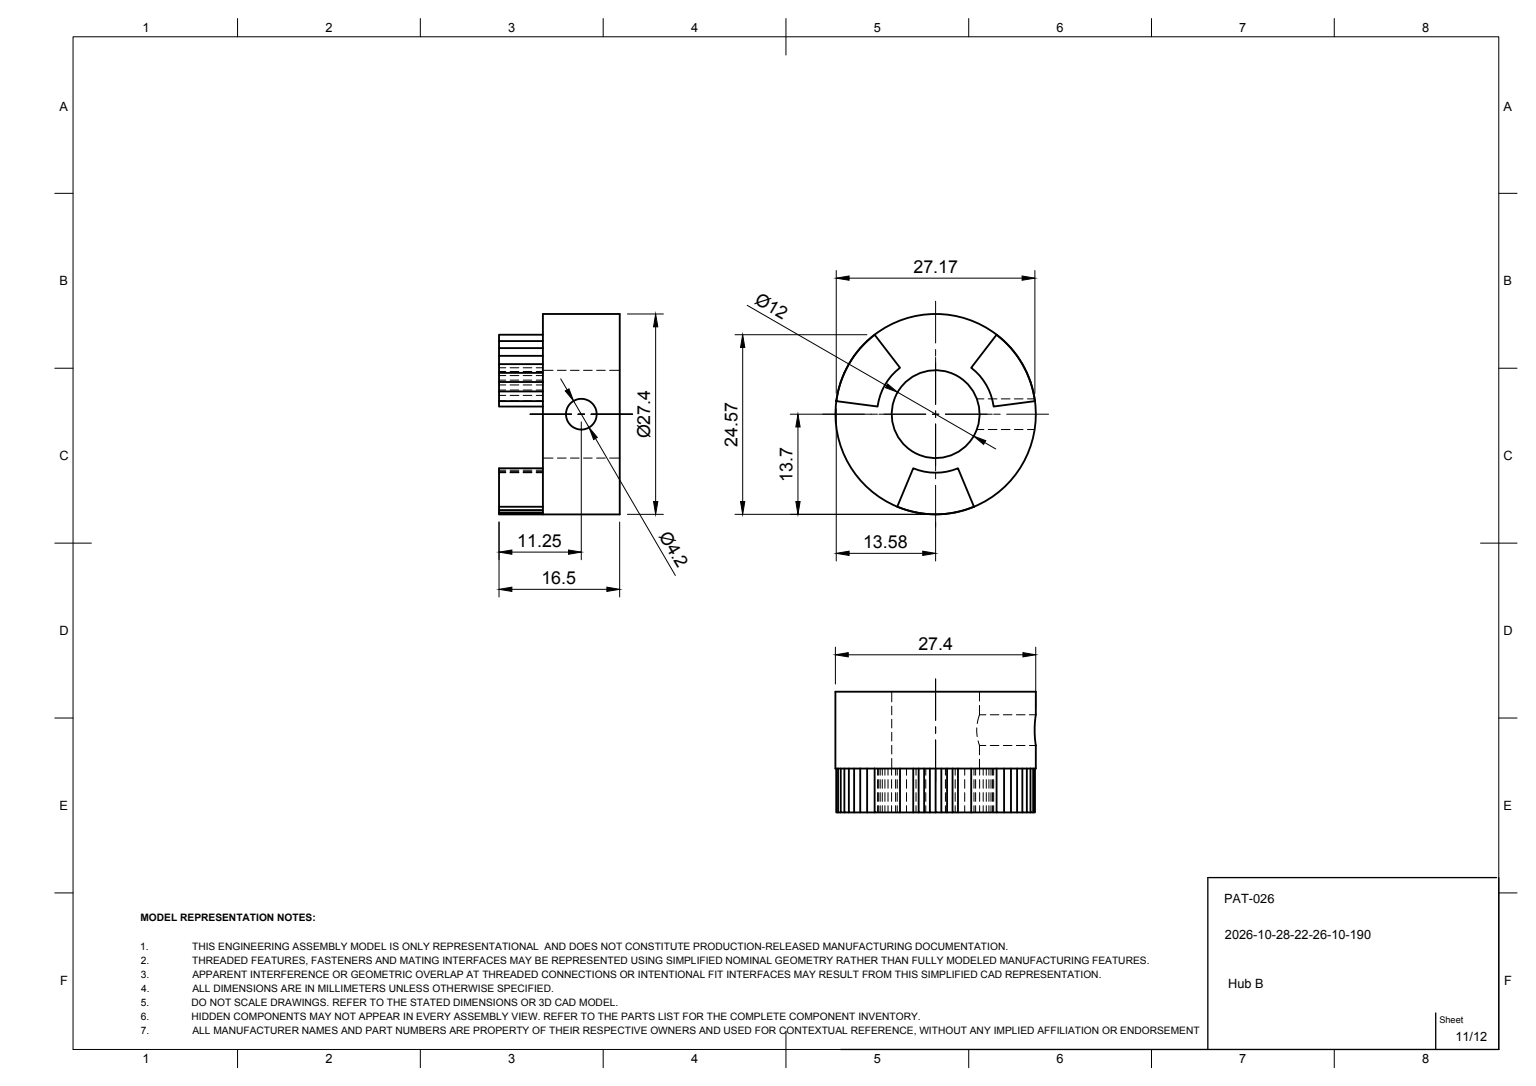
ISO-10303-21;
HEADER;
/* Generated by software containing ST-Developer
 * from STEP Tools, Inc. (www.steptools.com) 
 */

FILE_DESCRIPTION(
/* description */ ('PAT-026'),
/* implementation_level */ '2;1');

FILE_NAME(
/* name */ 'Hub B.step',
/* time_stamp */ '2026-10-28T22:25:58-07:00',
/* author */ (''),
/* organization */ (''),
/* preprocessor_version */ 'ST-DEVELOPER v20.2',
/* originating_system */ 'Autodesk Translation Framework v15.17.0.0',
/* authorisation */ '');

FILE_SCHEMA (('AUTOMOTIVE_DESIGN { 1 0 10303 214 3 1 1 }'));
ENDSEC;

DATA;
#10=MECHANICAL_DESIGN_GEOMETRIC_PRESENTATION_REPRESENTATION('',(#149),#12343);
#100=B_SPLINE_CURVE_WITH_KNOTS('',3,(#10943,#10944,#10945,#10946,#10947,
#10948,#10949,#10950,#10951,#10952,#10953,#10954,#10955,#10956,#10957,#10958,
#10959,#10960),.UNSPECIFIED.,.F.,.F.,(4,2,2,2,2,2,2,2,4),(0.,0.0798638474423531,
0.159727694884706,0.239545993340072,0.319364291795438,0.399182590250804,
0.47900088870617,0.558864736148523,0.638728583590876),.UNSPECIFIED.);
#101=B_SPLINE_CURVE_WITH_KNOTS('',3,(#10961,#10962,#10963,#10964,#10965,
#10966,#10967,#10968,#10969,#10970,#10971,#10972,#10973,#10974,#10975,#10976,
#10977,#10978),.UNSPECIFIED.,.F.,.F.,(4,2,2,2,2,2,2,2,4),(0.638728583590876,
0.718592431033229,0.798456278475583,0.878274576930949,0.958092875386314,
1.03791117384168,1.11772947229705,1.1975933197394,1.27745716718175),
 .UNSPECIFIED.);
#102=B_SPLINE_CURVE_WITH_KNOTS('',3,(#10982,#10983,#10984,#10985,#10986,
#10987,#10988,#10989,#10990,#10991,#10992,#10993,#10994,#10995,#10996,#10997,
#10998,#10999),.UNSPECIFIED.,.F.,.F.,(4,2,2,2,2,2,2,2,4),(0.,0.079239302416133,
0.158478604832266,0.237716399152057,0.316954193471848,0.39619198779164,
0.475429782111431,0.554669084527564,0.633908386943697),.UNSPECIFIED.);
#103=B_SPLINE_CURVE_WITH_KNOTS('',3,(#11000,#11001,#11002,#11003,#11004,
#11005,#11006,#11007,#11008,#11009,#11010,#11011,#11012,#11013,#11014,#11015,
#11016,#11017),.UNSPECIFIED.,.F.,.F.,(4,2,2,2,2,2,2,2,4),(0.633908386943697,
0.71314768935983,0.792386991775963,0.871624786095754,0.950862580415545,
1.03010037473534,1.10933816905513,1.18857747147126,1.26781677388739),
 .UNSPECIFIED.);
#127=SHAPE_REPRESENTATION_RELATIONSHIP('SRR','None',#12405,#138);
#138=ADVANCED_BREP_SHAPE_REPRESENTATION('',(#158),#12340);
#149=STYLED_ITEM('',(#12526),#158);
#158=MANIFOLD_SOLID_BREP('Body1',#7357);
#189=FACE_BOUND('',#1151,.T.);
#190=FACE_BOUND('',#1178,.T.);
#191=FACE_BOUND('',#1236,.T.);
#192=FACE_BOUND('',#1238,.T.);
#327=PLANE('',#7740);
#328=PLANE('',#7741);
#329=PLANE('',#7742);
#330=PLANE('',#7743);
#331=PLANE('',#7744);
#332=PLANE('',#7745);
#333=PLANE('',#7746);
#334=PLANE('',#7747);
#335=PLANE('',#7748);
#336=PLANE('',#7749);
#337=PLANE('',#7750);
#338=PLANE('',#7751);
#339=PLANE('',#7752);
#340=PLANE('',#7753);
#341=PLANE('',#7754);
#342=PLANE('',#7755);
#343=PLANE('',#7756);
#344=PLANE('',#7757);
#345=PLANE('',#7758);
#346=PLANE('',#7759);
#347=PLANE('',#7761);
#348=PLANE('',#7763);
#349=PLANE('',#7765);
#350=PLANE('',#7767);
#351=PLANE('',#7769);
#352=PLANE('',#7771);
#353=PLANE('',#7776);
#354=PLANE('',#7778);
#355=PLANE('',#7780);
#356=PLANE('',#7781);
#357=PLANE('',#7782);
#358=PLANE('',#7783);
#359=PLANE('',#7784);
#360=PLANE('',#7785);
#361=PLANE('',#7786);
#362=PLANE('',#7787);
#363=PLANE('',#7788);
#364=PLANE('',#7789);
#365=PLANE('',#7790);
#366=PLANE('',#7791);
#367=PLANE('',#7792);
#368=PLANE('',#7793);
#369=PLANE('',#7794);
#370=PLANE('',#7795);
#371=PLANE('',#7796);
#372=PLANE('',#7797);
#373=PLANE('',#7798);
#374=PLANE('',#7799);
#375=PLANE('',#7801);
#376=PLANE('',#7803);
#377=PLANE('',#7805);
#378=PLANE('',#7807);
#379=PLANE('',#7809);
#380=PLANE('',#7811);
#381=PLANE('',#7813);
#382=PLANE('',#7815);
#383=PLANE('',#7816);
#384=PLANE('',#7817);
#385=PLANE('',#7818);
#386=PLANE('',#7819);
#387=PLANE('',#7820);
#388=PLANE('',#7821);
#389=PLANE('',#7822);
#390=PLANE('',#7823);
#391=PLANE('',#7824);
#392=PLANE('',#7825);
#393=PLANE('',#7826);
#394=PLANE('',#7827);
#395=PLANE('',#7828);
#396=PLANE('',#7829);
#397=PLANE('',#7830);
#398=PLANE('',#7831);
#399=PLANE('',#7832);
#400=PLANE('',#7833);
#401=PLANE('',#7834);
#402=PLANE('',#7836);
#403=PLANE('',#7838);
#404=PLANE('',#7840);
#405=PLANE('',#7842);
#406=PLANE('',#7844);
#407=PLANE('',#7846);
#408=PLANE('',#7848);
#409=PLANE('',#7852);
#718=FACE_OUTER_BOUND('',#1149,.T.);
#719=FACE_OUTER_BOUND('',#1150,.T.);
#720=FACE_OUTER_BOUND('',#1152,.T.);
#721=FACE_OUTER_BOUND('',#1153,.T.);
#722=FACE_OUTER_BOUND('',#1154,.T.);
#723=FACE_OUTER_BOUND('',#1155,.T.);
#724=FACE_OUTER_BOUND('',#1156,.T.);
#725=FACE_OUTER_BOUND('',#1157,.T.);
#726=FACE_OUTER_BOUND('',#1158,.T.);
#727=FACE_OUTER_BOUND('',#1159,.T.);
#728=FACE_OUTER_BOUND('',#1160,.T.);
#729=FACE_OUTER_BOUND('',#1161,.T.);
#730=FACE_OUTER_BOUND('',#1162,.T.);
#731=FACE_OUTER_BOUND('',#1163,.T.);
#732=FACE_OUTER_BOUND('',#1164,.T.);
#733=FACE_OUTER_BOUND('',#1165,.T.);
#734=FACE_OUTER_BOUND('',#1166,.T.);
#735=FACE_OUTER_BOUND('',#1167,.T.);
#736=FACE_OUTER_BOUND('',#1168,.T.);
#737=FACE_OUTER_BOUND('',#1169,.T.);
#738=FACE_OUTER_BOUND('',#1170,.T.);
#739=FACE_OUTER_BOUND('',#1171,.T.);
#740=FACE_OUTER_BOUND('',#1172,.T.);
#741=FACE_OUTER_BOUND('',#1173,.T.);
#742=FACE_OUTER_BOUND('',#1174,.T.);
#743=FACE_OUTER_BOUND('',#1175,.T.);
#744=FACE_OUTER_BOUND('',#1176,.T.);
#745=FACE_OUTER_BOUND('',#1177,.T.);
#746=FACE_OUTER_BOUND('',#1179,.T.);
#747=FACE_OUTER_BOUND('',#1180,.T.);
#748=FACE_OUTER_BOUND('',#1181,.T.);
#749=FACE_OUTER_BOUND('',#1182,.T.);
#750=FACE_OUTER_BOUND('',#1183,.T.);
#751=FACE_OUTER_BOUND('',#1184,.T.);
#752=FACE_OUTER_BOUND('',#1185,.T.);
#753=FACE_OUTER_BOUND('',#1186,.T.);
#754=FACE_OUTER_BOUND('',#1187,.T.);
#755=FACE_OUTER_BOUND('',#1188,.T.);
#756=FACE_OUTER_BOUND('',#1189,.T.);
#757=FACE_OUTER_BOUND('',#1190,.T.);
#758=FACE_OUTER_BOUND('',#1191,.T.);
#759=FACE_OUTER_BOUND('',#1192,.T.);
#760=FACE_OUTER_BOUND('',#1193,.T.);
#761=FACE_OUTER_BOUND('',#1194,.T.);
#762=FACE_OUTER_BOUND('',#1195,.T.);
#763=FACE_OUTER_BOUND('',#1196,.T.);
#764=FACE_OUTER_BOUND('',#1197,.T.);
#765=FACE_OUTER_BOUND('',#1198,.T.);
#766=FACE_OUTER_BOUND('',#1199,.T.);
#767=FACE_OUTER_BOUND('',#1200,.T.);
#768=FACE_OUTER_BOUND('',#1201,.T.);
#769=FACE_OUTER_BOUND('',#1202,.T.);
#770=FACE_OUTER_BOUND('',#1203,.T.);
#771=FACE_OUTER_BOUND('',#1204,.T.);
#772=FACE_OUTER_BOUND('',#1205,.T.);
#773=FACE_OUTER_BOUND('',#1206,.T.);
#774=FACE_OUTER_BOUND('',#1207,.T.);
#775=FACE_OUTER_BOUND('',#1208,.T.);
#776=FACE_OUTER_BOUND('',#1209,.T.);
#777=FACE_OUTER_BOUND('',#1210,.T.);
#778=FACE_OUTER_BOUND('',#1211,.T.);
#779=FACE_OUTER_BOUND('',#1212,.T.);
#780=FACE_OUTER_BOUND('',#1213,.T.);
#781=FACE_OUTER_BOUND('',#1214,.T.);
#782=FACE_OUTER_BOUND('',#1215,.T.);
#783=FACE_OUTER_BOUND('',#1216,.T.);
#784=FACE_OUTER_BOUND('',#1217,.T.);
#785=FACE_OUTER_BOUND('',#1218,.T.);
#786=FACE_OUTER_BOUND('',#1219,.T.);
#787=FACE_OUTER_BOUND('',#1220,.T.);
#788=FACE_OUTER_BOUND('',#1221,.T.);
#789=FACE_OUTER_BOUND('',#1222,.T.);
#790=FACE_OUTER_BOUND('',#1223,.T.);
#791=FACE_OUTER_BOUND('',#1224,.T.);
#792=FACE_OUTER_BOUND('',#1225,.T.);
#793=FACE_OUTER_BOUND('',#1226,.T.);
#794=FACE_OUTER_BOUND('',#1227,.T.);
#795=FACE_OUTER_BOUND('',#1228,.T.);
#796=FACE_OUTER_BOUND('',#1229,.T.);
#797=FACE_OUTER_BOUND('',#1230,.T.);
#798=FACE_OUTER_BOUND('',#1231,.T.);
#799=FACE_OUTER_BOUND('',#1232,.T.);
#800=FACE_OUTER_BOUND('',#1233,.T.);
#801=FACE_OUTER_BOUND('',#1234,.T.);
#802=FACE_OUTER_BOUND('',#1235,.T.);
#803=FACE_OUTER_BOUND('',#1237,.T.);
#1149=EDGE_LOOP('',(#5633,#5634,#5635,#5636,#5637,#5638));
#1150=EDGE_LOOP('',(#5639,#5640,#5641,#5642));
#1151=EDGE_LOOP('',(#5643,#5644));
#1152=EDGE_LOOP('',(#5645,#5646,#5647,#5648));
#1153=EDGE_LOOP('',(#5649,#5650,#5651,#5652));
#1154=EDGE_LOOP('',(#5653,#5654,#5655,#5656));
#1155=EDGE_LOOP('',(#5657,#5658,#5659,#5660));
#1156=EDGE_LOOP('',(#5661,#5662,#5663,#5664));
#1157=EDGE_LOOP('',(#5665,#5666,#5667,#5668));
#1158=EDGE_LOOP('',(#5669,#5670,#5671,#5672));
#1159=EDGE_LOOP('',(#5673,#5674,#5675,#5676));
#1160=EDGE_LOOP('',(#5677,#5678,#5679,#5680));
#1161=EDGE_LOOP('',(#5681,#5682,#5683,#5684));
#1162=EDGE_LOOP('',(#5685,#5686,#5687,#5688));
#1163=EDGE_LOOP('',(#5689,#5690,#5691,#5692));
#1164=EDGE_LOOP('',(#5693,#5694,#5695,#5696));
#1165=EDGE_LOOP('',(#5697,#5698,#5699,#5700));
#1166=EDGE_LOOP('',(#5701,#5702,#5703,#5704));
#1167=EDGE_LOOP('',(#5705,#5706,#5707,#5708));
#1168=EDGE_LOOP('',(#5709,#5710,#5711,#5712));
#1169=EDGE_LOOP('',(#5713,#5714,#5715,#5716));
#1170=EDGE_LOOP('',(#5717,#5718,#5719,#5720,#5721,#5722,#5723,#5724,#5725,
#5726,#5727,#5728,#5729,#5730,#5731,#5732,#5733,#5734));
#1171=EDGE_LOOP('',(#5735,#5736));
#1172=EDGE_LOOP('',(#5737,#5738));
#1173=EDGE_LOOP('',(#5739,#5740));
#1174=EDGE_LOOP('',(#5741,#5742));
#1175=EDGE_LOOP('',(#5743,#5744));
#1176=EDGE_LOOP('',(#5745,#5746));
#1177=EDGE_LOOP('',(#5747,#5748,#5749,#5750,#5751,#5752,#5753,#5754,#5755,
#5756,#5757,#5758,#5759,#5760,#5761,#5762,#5763,#5764,#5765,#5766,#5767,
#5768,#5769,#5770,#5771,#5772,#5773,#5774,#5775,#5776,#5777,#5778,#5779,
#5780));
#1178=EDGE_LOOP('',(#5781));
#1179=EDGE_LOOP('',(#5782,#5783));
#1180=EDGE_LOOP('',(#5784,#5785));
#1181=EDGE_LOOP('',(#5786,#5787,#5788,#5789));
#1182=EDGE_LOOP('',(#5790,#5791,#5792,#5793));
#1183=EDGE_LOOP('',(#5794,#5795,#5796,#5797));
#1184=EDGE_LOOP('',(#5798,#5799,#5800,#5801));
#1185=EDGE_LOOP('',(#5802,#5803,#5804,#5805));
#1186=EDGE_LOOP('',(#5806,#5807,#5808,#5809));
#1187=EDGE_LOOP('',(#5810,#5811,#5812,#5813));
#1188=EDGE_LOOP('',(#5814,#5815,#5816,#5817));
#1189=EDGE_LOOP('',(#5818,#5819,#5820,#5821));
#1190=EDGE_LOOP('',(#5822,#5823,#5824,#5825));
#1191=EDGE_LOOP('',(#5826,#5827,#5828,#5829));
#1192=EDGE_LOOP('',(#5830,#5831,#5832,#5833));
#1193=EDGE_LOOP('',(#5834,#5835,#5836,#5837));
#1194=EDGE_LOOP('',(#5838,#5839,#5840,#5841));
#1195=EDGE_LOOP('',(#5842,#5843,#5844,#5845));
#1196=EDGE_LOOP('',(#5846,#5847,#5848,#5849));
#1197=EDGE_LOOP('',(#5850,#5851,#5852,#5853));
#1198=EDGE_LOOP('',(#5854,#5855,#5856,#5857));
#1199=EDGE_LOOP('',(#5858,#5859,#5860,#5861,#5862,#5863,#5864,#5865,#5866,
#5867,#5868,#5869,#5870,#5871,#5872,#5873,#5874,#5875));
#1200=EDGE_LOOP('',(#5876,#5877));
#1201=EDGE_LOOP('',(#5878,#5879));
#1202=EDGE_LOOP('',(#5880,#5881));
#1203=EDGE_LOOP('',(#5882,#5883));
#1204=EDGE_LOOP('',(#5884,#5885));
#1205=EDGE_LOOP('',(#5886,#5887));
#1206=EDGE_LOOP('',(#5888,#5889));
#1207=EDGE_LOOP('',(#5890,#5891));
#1208=EDGE_LOOP('',(#5892,#5893,#5894,#5895));
#1209=EDGE_LOOP('',(#5896,#5897,#5898,#5899));
#1210=EDGE_LOOP('',(#5900,#5901,#5902,#5903));
#1211=EDGE_LOOP('',(#5904,#5905,#5906,#5907));
#1212=EDGE_LOOP('',(#5908,#5909,#5910,#5911));
#1213=EDGE_LOOP('',(#5912,#5913,#5914,#5915));
#1214=EDGE_LOOP('',(#5916,#5917,#5918,#5919));
#1215=EDGE_LOOP('',(#5920,#5921,#5922,#5923));
#1216=EDGE_LOOP('',(#5924,#5925,#5926,#5927));
#1217=EDGE_LOOP('',(#5928,#5929,#5930,#5931));
#1218=EDGE_LOOP('',(#5932,#5933,#5934,#5935));
#1219=EDGE_LOOP('',(#5936,#5937,#5938,#5939));
#1220=EDGE_LOOP('',(#5940,#5941,#5942,#5943));
#1221=EDGE_LOOP('',(#5944,#5945,#5946,#5947));
#1222=EDGE_LOOP('',(#5948,#5949,#5950,#5951));
#1223=EDGE_LOOP('',(#5952,#5953,#5954,#5955));
#1224=EDGE_LOOP('',(#5956,#5957,#5958,#5959));
#1225=EDGE_LOOP('',(#5960,#5961,#5962,#5963));
#1226=EDGE_LOOP('',(#5964,#5965,#5966,#5967,#5968,#5969,#5970,#5971,#5972,
#5973,#5974,#5975,#5976,#5977,#5978,#5979,#5980,#5981));
#1227=EDGE_LOOP('',(#5982,#5983));
#1228=EDGE_LOOP('',(#5984,#5985));
#1229=EDGE_LOOP('',(#5986,#5987));
#1230=EDGE_LOOP('',(#5988,#5989));
#1231=EDGE_LOOP('',(#5990,#5991));
#1232=EDGE_LOOP('',(#5992,#5993));
#1233=EDGE_LOOP('',(#5994,#5995));
#1234=EDGE_LOOP('',(#5996,#5997));
#1235=EDGE_LOOP('',(#5998,#5999,#6000,#6001,#6002,#6003,#6004,#6005,#6006,
#6007,#6008,#6009,#6010,#6011,#6012,#6013,#6014,#6015,#6016,#6017,#6018,
#6019,#6020,#6021,#6022,#6023,#6024,#6025,#6026,#6027,#6028));
#1236=EDGE_LOOP('',(#6029,#6030));
#1237=EDGE_LOOP('',(#6031));
#1238=EDGE_LOOP('',(#6032));
#1676=LINE('',#10980,#2548);
#1677=LINE('',#11022,#2549);
#1678=LINE('',#11027,#2550);
#1679=LINE('',#11029,#2551);
#1680=LINE('',#11031,#2552);
#1681=LINE('',#11032,#2553);
#1682=LINE('',#11035,#2554);
#1683=LINE('',#11037,#2555);
#1684=LINE('',#11038,#2556);
#1685=LINE('',#11041,#2557);
#1686=LINE('',#11043,#2558);
#1687=LINE('',#11044,#2559);
#1688=LINE('',#11047,#2560);
#1689=LINE('',#11049,#2561);
#1690=LINE('',#11050,#2562);
#1691=LINE('',#11053,#2563);
#1692=LINE('',#11055,#2564);
#1693=LINE('',#11056,#2565);
#1694=LINE('',#11059,#2566);
#1695=LINE('',#11061,#2567);
#1696=LINE('',#11062,#2568);
#1697=LINE('',#11065,#2569);
#1698=LINE('',#11067,#2570);
#1699=LINE('',#11068,#2571);
#1700=LINE('',#11071,#2572);
#1701=LINE('',#11073,#2573);
#1702=LINE('',#11074,#2574);
#1703=LINE('',#11077,#2575);
#1704=LINE('',#11079,#2576);
#1705=LINE('',#11080,#2577);
#1706=LINE('',#11083,#2578);
#1707=LINE('',#11085,#2579);
#1708=LINE('',#11086,#2580);
#1709=LINE('',#11089,#2581);
#1710=LINE('',#11091,#2582);
#1711=LINE('',#11092,#2583);
#1712=LINE('',#11095,#2584);
#1713=LINE('',#11097,#2585);
#1714=LINE('',#11098,#2586);
#1715=LINE('',#11101,#2587);
#1716=LINE('',#11103,#2588);
#1717=LINE('',#11104,#2589);
#1718=LINE('',#11107,#2590);
#1719=LINE('',#11109,#2591);
#1720=LINE('',#11110,#2592);
#1721=LINE('',#11113,#2593);
#1722=LINE('',#11115,#2594);
#1723=LINE('',#11116,#2595);
#1724=LINE('',#11119,#2596);
#1725=LINE('',#11121,#2597);
#1726=LINE('',#11122,#2598);
#1727=LINE('',#11125,#2599);
#1728=LINE('',#11127,#2600);
#1729=LINE('',#11128,#2601);
#1730=LINE('',#11130,#2602);
#1731=LINE('',#11131,#2603);
#1732=LINE('',#11151,#2604);
#1733=LINE('',#11153,#2605);
#1734=LINE('',#11155,#2606);
#1735=LINE('',#11157,#2607);
#1736=LINE('',#11159,#2608);
#1737=LINE('',#11161,#2609);
#1738=LINE('',#11163,#2610);
#1739=LINE('',#11165,#2611);
#1740=LINE('',#11167,#2612);
#1741=LINE('',#11169,#2613);
#1742=LINE('',#11173,#2614);
#1743=LINE('',#11175,#2615);
#1744=LINE('',#11177,#2616);
#1745=LINE('',#11179,#2617);
#1746=LINE('',#11181,#2618);
#1747=LINE('',#11183,#2619);
#1748=LINE('',#11185,#2620);
#1749=LINE('',#11187,#2621);
#1750=LINE('',#11189,#2622);
#1751=LINE('',#11191,#2623);
#1752=LINE('',#11200,#2624);
#1753=LINE('',#11201,#2625);
#1754=LINE('',#11202,#2626);
#1755=LINE('',#11205,#2627);
#1756=LINE('',#11206,#2628);
#1757=LINE('',#11209,#2629);
#1758=LINE('',#11210,#2630);
#1759=LINE('',#11213,#2631);
#1760=LINE('',#11214,#2632);
#1761=LINE('',#11217,#2633);
#1762=LINE('',#11218,#2634);
#1763=LINE('',#11221,#2635);
#1764=LINE('',#11222,#2636);
#1765=LINE('',#11225,#2637);
#1766=LINE('',#11226,#2638);
#1767=LINE('',#11229,#2639);
#1768=LINE('',#11230,#2640);
#1769=LINE('',#11233,#2641);
#1770=LINE('',#11234,#2642);
#1771=LINE('',#11237,#2643);
#1772=LINE('',#11239,#2644);
#1773=LINE('',#11240,#2645);
#1774=LINE('',#11243,#2646);
#1775=LINE('',#11245,#2647);
#1776=LINE('',#11246,#2648);
#1777=LINE('',#11249,#2649);
#1778=LINE('',#11251,#2650);
#1779=LINE('',#11252,#2651);
#1780=LINE('',#11255,#2652);
#1781=LINE('',#11257,#2653);
#1782=LINE('',#11258,#2654);
#1783=LINE('',#11261,#2655);
#1784=LINE('',#11263,#2656);
#1785=LINE('',#11264,#2657);
#1786=LINE('',#11267,#2658);
#1787=LINE('',#11269,#2659);
#1788=LINE('',#11270,#2660);
#1789=LINE('',#11273,#2661);
#1790=LINE('',#11275,#2662);
#1791=LINE('',#11276,#2663);
#1792=LINE('',#11279,#2664);
#1793=LINE('',#11280,#2665);
#1794=LINE('',#11281,#2666);
#1795=LINE('',#11283,#2667);
#1796=LINE('',#11304,#2668);
#1797=LINE('',#11305,#2669);
#1798=LINE('',#11306,#2670);
#1799=LINE('',#11309,#2671);
#1800=LINE('',#11310,#2672);
#1801=LINE('',#11313,#2673);
#1802=LINE('',#11314,#2674);
#1803=LINE('',#11317,#2675);
#1804=LINE('',#11318,#2676);
#1805=LINE('',#11321,#2677);
#1806=LINE('',#11322,#2678);
#1807=LINE('',#11325,#2679);
#1808=LINE('',#11326,#2680);
#1809=LINE('',#11329,#2681);
#1810=LINE('',#11330,#2682);
#1811=LINE('',#11333,#2683);
#1812=LINE('',#11334,#2684);
#1813=LINE('',#11337,#2685);
#1814=LINE('',#11338,#2686);
#1815=LINE('',#11341,#2687);
#1816=LINE('',#11343,#2688);
#1817=LINE('',#11344,#2689);
#1818=LINE('',#11347,#2690);
#1819=LINE('',#11349,#2691);
#1820=LINE('',#11350,#2692);
#1821=LINE('',#11353,#2693);
#1822=LINE('',#11355,#2694);
#1823=LINE('',#11356,#2695);
#1824=LINE('',#11359,#2696);
#1825=LINE('',#11361,#2697);
#1826=LINE('',#11362,#2698);
#1827=LINE('',#11365,#2699);
#1828=LINE('',#11367,#2700);
#1829=LINE('',#11368,#2701);
#1830=LINE('',#11371,#2702);
#1831=LINE('',#11373,#2703);
#1832=LINE('',#11374,#2704);
#1833=LINE('',#11377,#2705);
#1834=LINE('',#11379,#2706);
#1835=LINE('',#11380,#2707);
#1836=LINE('',#11383,#2708);
#1837=LINE('',#11384,#2709);
#1838=LINE('',#11385,#2710);
#1839=LINE('',#11387,#2711);
#1840=LINE('',#11408,#2712);
#2548=VECTOR('',#8838,0.21);
#2549=VECTOR('',#8843,0.6);
#2550=VECTOR('',#8848,1.);
#2551=VECTOR('',#8849,1.);
#2552=VECTOR('',#8850,1.);
#2553=VECTOR('',#8851,1.);
#2554=VECTOR('',#8854,1.);
#2555=VECTOR('',#8855,1.);
#2556=VECTOR('',#8856,1.);
#2557=VECTOR('',#8859,1.);
#2558=VECTOR('',#8860,1.);
#2559=VECTOR('',#8861,1.);
#2560=VECTOR('',#8864,1.);
#2561=VECTOR('',#8865,1.);
#2562=VECTOR('',#8866,1.);
#2563=VECTOR('',#8869,1.);
#2564=VECTOR('',#8870,1.);
#2565=VECTOR('',#8871,1.);
#2566=VECTOR('',#8874,1.);
#2567=VECTOR('',#8875,1.);
#2568=VECTOR('',#8876,1.);
#2569=VECTOR('',#8879,1.);
#2570=VECTOR('',#8880,1.);
#2571=VECTOR('',#8881,1.);
#2572=VECTOR('',#8884,1.);
#2573=VECTOR('',#8885,1.);
#2574=VECTOR('',#8886,1.);
#2575=VECTOR('',#8889,1.);
#2576=VECTOR('',#8890,1.);
#2577=VECTOR('',#8891,1.);
#2578=VECTOR('',#8894,1.);
#2579=VECTOR('',#8895,1.);
#2580=VECTOR('',#8896,1.);
#2581=VECTOR('',#8899,1.);
#2582=VECTOR('',#8900,1.);
#2583=VECTOR('',#8901,1.);
#2584=VECTOR('',#8904,1.);
#2585=VECTOR('',#8905,1.);
#2586=VECTOR('',#8906,1.);
#2587=VECTOR('',#8909,1.);
#2588=VECTOR('',#8910,1.);
#2589=VECTOR('',#8911,1.);
#2590=VECTOR('',#8914,1.);
#2591=VECTOR('',#8915,1.);
#2592=VECTOR('',#8916,1.);
#2593=VECTOR('',#8919,1.);
#2594=VECTOR('',#8920,1.);
#2595=VECTOR('',#8921,1.);
#2596=VECTOR('',#8924,1.);
#2597=VECTOR('',#8925,1.);
#2598=VECTOR('',#8926,1.);
#2599=VECTOR('',#8929,1.);
#2600=VECTOR('',#8930,1.);
#2601=VECTOR('',#8931,1.);
#2602=VECTOR('',#8934,1.);
#2603=VECTOR('',#8935,1.);
#2604=VECTOR('',#8968,1.);
#2605=VECTOR('',#8969,1.);
#2606=VECTOR('',#8970,1.);
#2607=VECTOR('',#8971,1.);
#2608=VECTOR('',#8972,1.);
#2609=VECTOR('',#8973,1.);
#2610=VECTOR('',#8974,1.);
#2611=VECTOR('',#8975,1.);
#2612=VECTOR('',#8976,1.);
#2613=VECTOR('',#8977,1.);
#2614=VECTOR('',#8980,1.);
#2615=VECTOR('',#8981,1.);
#2616=VECTOR('',#8982,1.);
#2617=VECTOR('',#8983,1.);
#2618=VECTOR('',#8984,1.);
#2619=VECTOR('',#8985,1.);
#2620=VECTOR('',#8986,1.);
#2621=VECTOR('',#8987,1.);
#2622=VECTOR('',#8988,1.);
#2623=VECTOR('',#8989,1.);
#2624=VECTOR('',#9002,1.);
#2625=VECTOR('',#9003,1.);
#2626=VECTOR('',#9004,1.);
#2627=VECTOR('',#9007,1.);
#2628=VECTOR('',#9008,1.);
#2629=VECTOR('',#9011,1.);
#2630=VECTOR('',#9012,1.);
#2631=VECTOR('',#9015,1.);
#2632=VECTOR('',#9016,1.);
#2633=VECTOR('',#9019,1.);
#2634=VECTOR('',#9020,1.);
#2635=VECTOR('',#9023,1.);
#2636=VECTOR('',#9024,1.);
#2637=VECTOR('',#9027,1.);
#2638=VECTOR('',#9028,1.);
#2639=VECTOR('',#9031,1.);
#2640=VECTOR('',#9032,1.);
#2641=VECTOR('',#9035,1.);
#2642=VECTOR('',#9036,1.);
#2643=VECTOR('',#9039,1.);
#2644=VECTOR('',#9040,1.);
#2645=VECTOR('',#9041,1.);
#2646=VECTOR('',#9044,1.);
#2647=VECTOR('',#9045,1.);
#2648=VECTOR('',#9046,1.);
#2649=VECTOR('',#9049,1.);
#2650=VECTOR('',#9050,1.);
#2651=VECTOR('',#9051,1.);
#2652=VECTOR('',#9054,1.);
#2653=VECTOR('',#9055,1.);
#2654=VECTOR('',#9056,1.);
#2655=VECTOR('',#9059,1.);
#2656=VECTOR('',#9060,1.);
#2657=VECTOR('',#9061,1.);
#2658=VECTOR('',#9064,1.);
#2659=VECTOR('',#9065,1.);
#2660=VECTOR('',#9066,1.);
#2661=VECTOR('',#9069,1.);
#2662=VECTOR('',#9070,1.);
#2663=VECTOR('',#9071,1.);
#2664=VECTOR('',#9074,1.);
#2665=VECTOR('',#9075,1.);
#2666=VECTOR('',#9076,1.);
#2667=VECTOR('',#9079,1.);
#2668=VECTOR('',#9116,1.);
#2669=VECTOR('',#9117,1.);
#2670=VECTOR('',#9118,1.);
#2671=VECTOR('',#9121,1.);
#2672=VECTOR('',#9122,1.);
#2673=VECTOR('',#9125,1.);
#2674=VECTOR('',#9126,1.);
#2675=VECTOR('',#9129,1.);
#2676=VECTOR('',#9130,1.);
#2677=VECTOR('',#9133,1.);
#2678=VECTOR('',#9134,1.);
#2679=VECTOR('',#9137,1.);
#2680=VECTOR('',#9138,1.);
#2681=VECTOR('',#9141,1.);
#2682=VECTOR('',#9142,1.);
#2683=VECTOR('',#9145,1.);
#2684=VECTOR('',#9146,1.);
#2685=VECTOR('',#9149,1.);
#2686=VECTOR('',#9150,1.);
#2687=VECTOR('',#9153,1.);
#2688=VECTOR('',#9154,1.);
#2689=VECTOR('',#9155,1.);
#2690=VECTOR('',#9158,1.);
#2691=VECTOR('',#9159,1.);
#2692=VECTOR('',#9160,1.);
#2693=VECTOR('',#9163,1.);
#2694=VECTOR('',#9164,1.);
#2695=VECTOR('',#9165,1.);
#2696=VECTOR('',#9168,1.);
#2697=VECTOR('',#9169,1.);
#2698=VECTOR('',#9170,1.);
#2699=VECTOR('',#9173,1.);
#2700=VECTOR('',#9174,1.);
#2701=VECTOR('',#9175,1.);
#2702=VECTOR('',#9178,1.);
#2703=VECTOR('',#9179,1.);
#2704=VECTOR('',#9180,1.);
#2705=VECTOR('',#9183,1.);
#2706=VECTOR('',#9184,1.);
#2707=VECTOR('',#9185,1.);
#2708=VECTOR('',#9188,1.);
#2709=VECTOR('',#9189,1.);
#2710=VECTOR('',#9190,1.);
#2711=VECTOR('',#9193,1.);
#2712=VECTOR('',#9232,1.37);
#3214=CIRCLE('',#7738,0.6);
#3215=CIRCLE('',#7739,0.6);
#3216=CIRCLE('',#7760,1.37);
#3217=CIRCLE('',#7762,1.37);
#3218=CIRCLE('',#7764,1.37);
#3219=CIRCLE('',#7766,1.37);
#3220=CIRCLE('',#7768,1.37);
#3221=CIRCLE('',#7770,1.37);
#3222=CIRCLE('',#7772,1.37);
#3223=CIRCLE('',#7773,1.37);
#3224=CIRCLE('',#7774,1.37);
#3225=CIRCLE('',#7775,1.37);
#3226=CIRCLE('',#7777,1.37);
#3227=CIRCLE('',#7779,1.37);
#3228=CIRCLE('',#7800,1.37);
#3229=CIRCLE('',#7802,1.37);
#3230=CIRCLE('',#7804,1.37);
#3231=CIRCLE('',#7806,1.37);
#3232=CIRCLE('',#7808,1.37);
#3233=CIRCLE('',#7810,1.37);
#3234=CIRCLE('',#7812,1.37);
#3235=CIRCLE('',#7814,1.37);
#3236=CIRCLE('',#7835,1.37);
#3237=CIRCLE('',#7837,1.37);
#3238=CIRCLE('',#7839,1.37);
#3239=CIRCLE('',#7841,1.37);
#3240=CIRCLE('',#7843,1.37);
#3241=CIRCLE('',#7845,1.37);
#3242=CIRCLE('',#7847,1.37);
#3243=CIRCLE('',#7849,1.37);
#3244=CIRCLE('',#7851,1.37);
#3485=VERTEX_POINT('',#10941);
#3486=VERTEX_POINT('',#10942);
#3487=VERTEX_POINT('',#10979);
#3488=VERTEX_POINT('',#10981);
#3489=VERTEX_POINT('',#11019);
#3490=VERTEX_POINT('',#11021);
#3491=VERTEX_POINT('',#11025);
#3492=VERTEX_POINT('',#11026);
#3493=VERTEX_POINT('',#11028);
#3494=VERTEX_POINT('',#11030);
#3495=VERTEX_POINT('',#11034);
#3496=VERTEX_POINT('',#11036);
#3497=VERTEX_POINT('',#11040);
#3498=VERTEX_POINT('',#11042);
#3499=VERTEX_POINT('',#11046);
#3500=VERTEX_POINT('',#11048);
#3501=VERTEX_POINT('',#11052);
#3502=VERTEX_POINT('',#11054);
#3503=VERTEX_POINT('',#11058);
#3504=VERTEX_POINT('',#11060);
#3505=VERTEX_POINT('',#11064);
#3506=VERTEX_POINT('',#11066);
#3507=VERTEX_POINT('',#11070);
#3508=VERTEX_POINT('',#11072);
#3509=VERTEX_POINT('',#11076);
#3510=VERTEX_POINT('',#11078);
#3511=VERTEX_POINT('',#11082);
#3512=VERTEX_POINT('',#11084);
#3513=VERTEX_POINT('',#11088);
#3514=VERTEX_POINT('',#11090);
#3515=VERTEX_POINT('',#11094);
#3516=VERTEX_POINT('',#11096);
#3517=VERTEX_POINT('',#11100);
#3518=VERTEX_POINT('',#11102);
#3519=VERTEX_POINT('',#11106);
#3520=VERTEX_POINT('',#11108);
#3521=VERTEX_POINT('',#11112);
#3522=VERTEX_POINT('',#11114);
#3523=VERTEX_POINT('',#11118);
#3524=VERTEX_POINT('',#11120);
#3525=VERTEX_POINT('',#11124);
#3526=VERTEX_POINT('',#11126);
#3527=VERTEX_POINT('',#11146);
#3528=VERTEX_POINT('',#11148);
#3529=VERTEX_POINT('',#11150);
#3530=VERTEX_POINT('',#11152);
#3531=VERTEX_POINT('',#11154);
#3532=VERTEX_POINT('',#11156);
#3533=VERTEX_POINT('',#11158);
#3534=VERTEX_POINT('',#11160);
#3535=VERTEX_POINT('',#11162);
#3536=VERTEX_POINT('',#11164);
#3537=VERTEX_POINT('',#11166);
#3538=VERTEX_POINT('',#11168);
#3539=VERTEX_POINT('',#11170);
#3540=VERTEX_POINT('',#11172);
#3541=VERTEX_POINT('',#11174);
#3542=VERTEX_POINT('',#11176);
#3543=VERTEX_POINT('',#11178);
#3544=VERTEX_POINT('',#11180);
#3545=VERTEX_POINT('',#11182);
#3546=VERTEX_POINT('',#11184);
#3547=VERTEX_POINT('',#11186);
#3548=VERTEX_POINT('',#11188);
#3549=VERTEX_POINT('',#11190);
#3550=VERTEX_POINT('',#11198);
#3551=VERTEX_POINT('',#11199);
#3552=VERTEX_POINT('',#11204);
#3553=VERTEX_POINT('',#11208);
#3554=VERTEX_POINT('',#11212);
#3555=VERTEX_POINT('',#11216);
#3556=VERTEX_POINT('',#11220);
#3557=VERTEX_POINT('',#11224);
#3558=VERTEX_POINT('',#11228);
#3559=VERTEX_POINT('',#11232);
#3560=VERTEX_POINT('',#11236);
#3561=VERTEX_POINT('',#11238);
#3562=VERTEX_POINT('',#11242);
#3563=VERTEX_POINT('',#11244);
#3564=VERTEX_POINT('',#11248);
#3565=VERTEX_POINT('',#11250);
#3566=VERTEX_POINT('',#11254);
#3567=VERTEX_POINT('',#11256);
#3568=VERTEX_POINT('',#11260);
#3569=VERTEX_POINT('',#11262);
#3570=VERTEX_POINT('',#11266);
#3571=VERTEX_POINT('',#11268);
#3572=VERTEX_POINT('',#11272);
#3573=VERTEX_POINT('',#11274);
#3574=VERTEX_POINT('',#11278);
#3575=VERTEX_POINT('',#11302);
#3576=VERTEX_POINT('',#11303);
#3577=VERTEX_POINT('',#11308);
#3578=VERTEX_POINT('',#11312);
#3579=VERTEX_POINT('',#11316);
#3580=VERTEX_POINT('',#11320);
#3581=VERTEX_POINT('',#11324);
#3582=VERTEX_POINT('',#11328);
#3583=VERTEX_POINT('',#11332);
#3584=VERTEX_POINT('',#11336);
#3585=VERTEX_POINT('',#11340);
#3586=VERTEX_POINT('',#11342);
#3587=VERTEX_POINT('',#11346);
#3588=VERTEX_POINT('',#11348);
#3589=VERTEX_POINT('',#11352);
#3590=VERTEX_POINT('',#11354);
#3591=VERTEX_POINT('',#11358);
#3592=VERTEX_POINT('',#11360);
#3593=VERTEX_POINT('',#11364);
#3594=VERTEX_POINT('',#11366);
#3595=VERTEX_POINT('',#11370);
#3596=VERTEX_POINT('',#11372);
#3597=VERTEX_POINT('',#11376);
#3598=VERTEX_POINT('',#11378);
#3599=VERTEX_POINT('',#11382);
#3600=VERTEX_POINT('',#11406);
#4260=EDGE_CURVE('',#3485,#3486,#100,.T.);
#4261=EDGE_CURVE('',#3486,#3485,#101,.T.);
#4262=EDGE_CURVE('',#3486,#3487,#1676,.T.);
#4263=EDGE_CURVE('',#3488,#3487,#102,.T.);
#4264=EDGE_CURVE('',#3487,#3488,#103,.T.);
#4265=EDGE_CURVE('',#3489,#3489,#3214,.T.);
#4266=EDGE_CURVE('',#3489,#3490,#1677,.T.);
#4267=EDGE_CURVE('',#3490,#3490,#3215,.T.);
#4268=EDGE_CURVE('',#3491,#3492,#1678,.T.);
#4269=EDGE_CURVE('',#3492,#3493,#1679,.T.);
#4270=EDGE_CURVE('',#3494,#3493,#1680,.T.);
#4271=EDGE_CURVE('',#3491,#3494,#1681,.T.);
#4272=EDGE_CURVE('',#3495,#3491,#1682,.T.);
#4273=EDGE_CURVE('',#3496,#3494,#1683,.T.);
#4274=EDGE_CURVE('',#3495,#3496,#1684,.T.);
#4275=EDGE_CURVE('',#3497,#3495,#1685,.T.);
#4276=EDGE_CURVE('',#3498,#3496,#1686,.T.);
#4277=EDGE_CURVE('',#3497,#3498,#1687,.T.);
#4278=EDGE_CURVE('',#3499,#3497,#1688,.T.);
#4279=EDGE_CURVE('',#3500,#3498,#1689,.T.);
#4280=EDGE_CURVE('',#3499,#3500,#1690,.T.);
#4281=EDGE_CURVE('',#3501,#3499,#1691,.T.);
#4282=EDGE_CURVE('',#3502,#3500,#1692,.T.);
#4283=EDGE_CURVE('',#3501,#3502,#1693,.T.);
#4284=EDGE_CURVE('',#3503,#3501,#1694,.T.);
#4285=EDGE_CURVE('',#3504,#3502,#1695,.T.);
#4286=EDGE_CURVE('',#3503,#3504,#1696,.T.);
#4287=EDGE_CURVE('',#3505,#3503,#1697,.T.);
#4288=EDGE_CURVE('',#3506,#3504,#1698,.T.);
#4289=EDGE_CURVE('',#3505,#3506,#1699,.T.);
#4290=EDGE_CURVE('',#3507,#3505,#1700,.T.);
#4291=EDGE_CURVE('',#3508,#3506,#1701,.T.);
#4292=EDGE_CURVE('',#3507,#3508,#1702,.T.);
#4293=EDGE_CURVE('',#3509,#3507,#1703,.T.);
#4294=EDGE_CURVE('',#3510,#3508,#1704,.T.);
#4295=EDGE_CURVE('',#3509,#3510,#1705,.T.);
#4296=EDGE_CURVE('',#3511,#3509,#1706,.T.);
#4297=EDGE_CURVE('',#3512,#3510,#1707,.T.);
#4298=EDGE_CURVE('',#3511,#3512,#1708,.T.);
#4299=EDGE_CURVE('',#3513,#3511,#1709,.T.);
#4300=EDGE_CURVE('',#3514,#3512,#1710,.T.);
#4301=EDGE_CURVE('',#3513,#3514,#1711,.T.);
#4302=EDGE_CURVE('',#3515,#3513,#1712,.T.);
#4303=EDGE_CURVE('',#3516,#3514,#1713,.T.);
#4304=EDGE_CURVE('',#3515,#3516,#1714,.T.);
#4305=EDGE_CURVE('',#3517,#3515,#1715,.T.);
#4306=EDGE_CURVE('',#3518,#3516,#1716,.T.);
#4307=EDGE_CURVE('',#3517,#3518,#1717,.T.);
#4308=EDGE_CURVE('',#3519,#3517,#1718,.T.);
#4309=EDGE_CURVE('',#3520,#3518,#1719,.T.);
#4310=EDGE_CURVE('',#3519,#3520,#1720,.T.);
#4311=EDGE_CURVE('',#3521,#3519,#1721,.T.);
#4312=EDGE_CURVE('',#3522,#3520,#1722,.T.);
#4313=EDGE_CURVE('',#3521,#3522,#1723,.T.);
#4314=EDGE_CURVE('',#3523,#3521,#1724,.T.);
#4315=EDGE_CURVE('',#3524,#3522,#1725,.T.);
#4316=EDGE_CURVE('',#3523,#3524,#1726,.T.);
#4317=EDGE_CURVE('',#3525,#3523,#1727,.T.);
#4318=EDGE_CURVE('',#3526,#3524,#1728,.T.);
#4319=EDGE_CURVE('',#3525,#3526,#1729,.T.);
#4320=EDGE_CURVE('',#3492,#3525,#1730,.T.);
#4321=EDGE_CURVE('',#3493,#3526,#1731,.T.);
#4322=EDGE_CURVE('',#3526,#3524,#3216,.T.);
#4323=EDGE_CURVE('',#3524,#3522,#3217,.T.);
#4324=EDGE_CURVE('',#3522,#3520,#3218,.T.);
#4325=EDGE_CURVE('',#3520,#3518,#3219,.T.);
#4326=EDGE_CURVE('',#3518,#3516,#3220,.T.);
#4327=EDGE_CURVE('',#3516,#3514,#3221,.T.);
#4328=EDGE_CURVE('',#3527,#3526,#3222,.T.);
#4329=EDGE_CURVE('',#3528,#3527,#3223,.T.);
#4330=EDGE_CURVE('',#3528,#3529,#1732,.T.);
#4331=EDGE_CURVE('',#3529,#3530,#1733,.T.);
#4332=EDGE_CURVE('',#3530,#3531,#1734,.T.);
#4333=EDGE_CURVE('',#3531,#3532,#1735,.T.);
#4334=EDGE_CURVE('',#3532,#3533,#1736,.T.);
#4335=EDGE_CURVE('',#3533,#3534,#1737,.T.);
#4336=EDGE_CURVE('',#3534,#3535,#1738,.T.);
#4337=EDGE_CURVE('',#3535,#3536,#1739,.T.);
#4338=EDGE_CURVE('',#3536,#3537,#1740,.T.);
#4339=EDGE_CURVE('',#3537,#3538,#1741,.T.);
#4340=EDGE_CURVE('',#3539,#3538,#3224,.T.);
#4341=EDGE_CURVE('',#3539,#3540,#1742,.T.);
#4342=EDGE_CURVE('',#3540,#3541,#1743,.T.);
#4343=EDGE_CURVE('',#3541,#3542,#1744,.T.);
#4344=EDGE_CURVE('',#3542,#3543,#1745,.T.);
#4345=EDGE_CURVE('',#3543,#3544,#1746,.T.);
#4346=EDGE_CURVE('',#3544,#3545,#1747,.T.);
#4347=EDGE_CURVE('',#3545,#3546,#1748,.T.);
#4348=EDGE_CURVE('',#3546,#3547,#1749,.T.);
#4349=EDGE_CURVE('',#3547,#3548,#1750,.T.);
#4350=EDGE_CURVE('',#3548,#3549,#1751,.T.);
#4351=EDGE_CURVE('',#3510,#3549,#3225,.T.);
#4352=EDGE_CURVE('',#3512,#3510,#3226,.T.);
#4353=EDGE_CURVE('',#3514,#3512,#3227,.T.);
#4354=EDGE_CURVE('',#3550,#3551,#1752,.T.);
#4355=EDGE_CURVE('',#3551,#3537,#1753,.T.);
#4356=EDGE_CURVE('',#3550,#3536,#1754,.T.);
#4357=EDGE_CURVE('',#3552,#3550,#1755,.T.);
#4358=EDGE_CURVE('',#3552,#3535,#1756,.T.);
#4359=EDGE_CURVE('',#3553,#3552,#1757,.T.);
#4360=EDGE_CURVE('',#3553,#3534,#1758,.T.);
#4361=EDGE_CURVE('',#3554,#3553,#1759,.T.);
#4362=EDGE_CURVE('',#3554,#3533,#1760,.T.);
#4363=EDGE_CURVE('',#3555,#3554,#1761,.T.);
#4364=EDGE_CURVE('',#3555,#3532,#1762,.T.);
#4365=EDGE_CURVE('',#3556,#3555,#1763,.T.);
#4366=EDGE_CURVE('',#3556,#3531,#1764,.T.);
#4367=EDGE_CURVE('',#3557,#3556,#1765,.T.);
#4368=EDGE_CURVE('',#3557,#3530,#1766,.T.);
#4369=EDGE_CURVE('',#3558,#3557,#1767,.T.);
#4370=EDGE_CURVE('',#3558,#3529,#1768,.T.);
#4371=EDGE_CURVE('',#3559,#3558,#1769,.T.);
#4372=EDGE_CURVE('',#3559,#3528,#1770,.T.);
#4373=EDGE_CURVE('',#3560,#3559,#1771,.T.);
#4374=EDGE_CURVE('',#3561,#3528,#1772,.T.);
#4375=EDGE_CURVE('',#3560,#3561,#1773,.T.);
#4376=EDGE_CURVE('',#3562,#3560,#1774,.T.);
#4377=EDGE_CURVE('',#3563,#3561,#1775,.T.);
#4378=EDGE_CURVE('',#3562,#3563,#1776,.T.);
#4379=EDGE_CURVE('',#3564,#3562,#1777,.T.);
#4380=EDGE_CURVE('',#3565,#3563,#1778,.T.);
#4381=EDGE_CURVE('',#3564,#3565,#1779,.T.);
#4382=EDGE_CURVE('',#3566,#3564,#1780,.T.);
#4383=EDGE_CURVE('',#3567,#3565,#1781,.T.);
#4384=EDGE_CURVE('',#3566,#3567,#1782,.T.);
#4385=EDGE_CURVE('',#3568,#3566,#1783,.T.);
#4386=EDGE_CURVE('',#3569,#3567,#1784,.T.);
#4387=EDGE_CURVE('',#3568,#3569,#1785,.T.);
#4388=EDGE_CURVE('',#3570,#3568,#1786,.T.);
#4389=EDGE_CURVE('',#3571,#3569,#1787,.T.);
#4390=EDGE_CURVE('',#3570,#3571,#1788,.T.);
#4391=EDGE_CURVE('',#3572,#3570,#1789,.T.);
#4392=EDGE_CURVE('',#3573,#3571,#1790,.T.);
#4393=EDGE_CURVE('',#3572,#3573,#1791,.T.);
#4394=EDGE_CURVE('',#3574,#3572,#1792,.T.);
#4395=EDGE_CURVE('',#3538,#3573,#1793,.T.);
#4396=EDGE_CURVE('',#3574,#3538,#1794,.T.);
#4397=EDGE_CURVE('',#3551,#3574,#1795,.T.);
#4398=EDGE_CURVE('',#3538,#3573,#3228,.T.);
#4399=EDGE_CURVE('',#3573,#3571,#3229,.T.);
#4400=EDGE_CURVE('',#3571,#3569,#3230,.T.);
#4401=EDGE_CURVE('',#3569,#3567,#3231,.T.);
#4402=EDGE_CURVE('',#3567,#3565,#3232,.T.);
#4403=EDGE_CURVE('',#3565,#3563,#3233,.T.);
#4404=EDGE_CURVE('',#3561,#3528,#3234,.T.);
#4405=EDGE_CURVE('',#3563,#3561,#3235,.T.);
#4406=EDGE_CURVE('',#3575,#3576,#1796,.T.);
#4407=EDGE_CURVE('',#3576,#3548,#1797,.T.);
#4408=EDGE_CURVE('',#3575,#3547,#1798,.T.);
#4409=EDGE_CURVE('',#3577,#3575,#1799,.T.);
#4410=EDGE_CURVE('',#3577,#3546,#1800,.T.);
#4411=EDGE_CURVE('',#3578,#3577,#1801,.T.);
#4412=EDGE_CURVE('',#3578,#3545,#1802,.T.);
#4413=EDGE_CURVE('',#3579,#3578,#1803,.T.);
#4414=EDGE_CURVE('',#3579,#3544,#1804,.T.);
#4415=EDGE_CURVE('',#3580,#3579,#1805,.T.);
#4416=EDGE_CURVE('',#3580,#3543,#1806,.T.);
#4417=EDGE_CURVE('',#3581,#3580,#1807,.T.);
#4418=EDGE_CURVE('',#3581,#3542,#1808,.T.);
#4419=EDGE_CURVE('',#3582,#3581,#1809,.T.);
#4420=EDGE_CURVE('',#3582,#3541,#1810,.T.);
#4421=EDGE_CURVE('',#3583,#3582,#1811,.T.);
#4422=EDGE_CURVE('',#3583,#3540,#1812,.T.);
#4423=EDGE_CURVE('',#3584,#3583,#1813,.T.);
#4424=EDGE_CURVE('',#3584,#3539,#1814,.T.);
#4425=EDGE_CURVE('',#3585,#3584,#1815,.T.);
#4426=EDGE_CURVE('',#3586,#3539,#1816,.T.);
#4427=EDGE_CURVE('',#3585,#3586,#1817,.T.);
#4428=EDGE_CURVE('',#3587,#3585,#1818,.T.);
#4429=EDGE_CURVE('',#3588,#3586,#1819,.T.);
#4430=EDGE_CURVE('',#3587,#3588,#1820,.T.);
#4431=EDGE_CURVE('',#3589,#3587,#1821,.T.);
#4432=EDGE_CURVE('',#3590,#3588,#1822,.T.);
#4433=EDGE_CURVE('',#3589,#3590,#1823,.T.);
#4434=EDGE_CURVE('',#3591,#3589,#1824,.T.);
#4435=EDGE_CURVE('',#3592,#3590,#1825,.T.);
#4436=EDGE_CURVE('',#3591,#3592,#1826,.T.);
#4437=EDGE_CURVE('',#3593,#3591,#1827,.T.);
#4438=EDGE_CURVE('',#3594,#3592,#1828,.T.);
#4439=EDGE_CURVE('',#3593,#3594,#1829,.T.);
#4440=EDGE_CURVE('',#3595,#3593,#1830,.T.);
#4441=EDGE_CURVE('',#3596,#3594,#1831,.T.);
#4442=EDGE_CURVE('',#3595,#3596,#1832,.T.);
#4443=EDGE_CURVE('',#3597,#3595,#1833,.T.);
#4444=EDGE_CURVE('',#3598,#3596,#1834,.T.);
#4445=EDGE_CURVE('',#3597,#3598,#1835,.T.);
#4446=EDGE_CURVE('',#3599,#3597,#1836,.T.);
#4447=EDGE_CURVE('',#3549,#3598,#1837,.T.);
#4448=EDGE_CURVE('',#3599,#3549,#1838,.T.);
#4449=EDGE_CURVE('',#3576,#3599,#1839,.T.);
#4450=EDGE_CURVE('',#3549,#3598,#3236,.T.);
#4451=EDGE_CURVE('',#3598,#3596,#3237,.T.);
#4452=EDGE_CURVE('',#3596,#3594,#3238,.T.);
#4453=EDGE_CURVE('',#3594,#3592,#3239,.T.);
#4454=EDGE_CURVE('',#3592,#3590,#3240,.T.);
#4455=EDGE_CURVE('',#3590,#3588,#3241,.T.);
#4456=EDGE_CURVE('',#3586,#3539,#3242,.T.);
#4457=EDGE_CURVE('',#3588,#3586,#3243,.T.);
#4458=EDGE_CURVE('',#3600,#3600,#3244,.T.);
#4459=EDGE_CURVE('',#3600,#3527,#1840,.T.);
#5633=ORIENTED_EDGE('',*,*,#4260,.F.);
#5634=ORIENTED_EDGE('',*,*,#4261,.F.);
#5635=ORIENTED_EDGE('',*,*,#4262,.T.);
#5636=ORIENTED_EDGE('',*,*,#4263,.F.);
#5637=ORIENTED_EDGE('',*,*,#4264,.F.);
#5638=ORIENTED_EDGE('',*,*,#4262,.F.);
#5639=ORIENTED_EDGE('',*,*,#4265,.F.);
#5640=ORIENTED_EDGE('',*,*,#4266,.T.);
#5641=ORIENTED_EDGE('',*,*,#4267,.F.);
#5642=ORIENTED_EDGE('',*,*,#4266,.F.);
#5643=ORIENTED_EDGE('',*,*,#4260,.T.);
#5644=ORIENTED_EDGE('',*,*,#4261,.T.);
#5645=ORIENTED_EDGE('',*,*,#4268,.T.);
#5646=ORIENTED_EDGE('',*,*,#4269,.T.);
#5647=ORIENTED_EDGE('',*,*,#4270,.F.);
#5648=ORIENTED_EDGE('',*,*,#4271,.F.);
#5649=ORIENTED_EDGE('',*,*,#4272,.T.);
#5650=ORIENTED_EDGE('',*,*,#4271,.T.);
#5651=ORIENTED_EDGE('',*,*,#4273,.F.);
#5652=ORIENTED_EDGE('',*,*,#4274,.F.);
#5653=ORIENTED_EDGE('',*,*,#4275,.T.);
#5654=ORIENTED_EDGE('',*,*,#4274,.T.);
#5655=ORIENTED_EDGE('',*,*,#4276,.F.);
#5656=ORIENTED_EDGE('',*,*,#4277,.F.);
#5657=ORIENTED_EDGE('',*,*,#4278,.T.);
#5658=ORIENTED_EDGE('',*,*,#4277,.T.);
#5659=ORIENTED_EDGE('',*,*,#4279,.F.);
#5660=ORIENTED_EDGE('',*,*,#4280,.F.);
#5661=ORIENTED_EDGE('',*,*,#4281,.T.);
#5662=ORIENTED_EDGE('',*,*,#4280,.T.);
#5663=ORIENTED_EDGE('',*,*,#4282,.F.);
#5664=ORIENTED_EDGE('',*,*,#4283,.F.);
#5665=ORIENTED_EDGE('',*,*,#4284,.T.);
#5666=ORIENTED_EDGE('',*,*,#4283,.T.);
#5667=ORIENTED_EDGE('',*,*,#4285,.F.);
#5668=ORIENTED_EDGE('',*,*,#4286,.F.);
#5669=ORIENTED_EDGE('',*,*,#4287,.T.);
#5670=ORIENTED_EDGE('',*,*,#4286,.T.);
#5671=ORIENTED_EDGE('',*,*,#4288,.F.);
#5672=ORIENTED_EDGE('',*,*,#4289,.F.);
#5673=ORIENTED_EDGE('',*,*,#4290,.T.);
#5674=ORIENTED_EDGE('',*,*,#4289,.T.);
#5675=ORIENTED_EDGE('',*,*,#4291,.F.);
#5676=ORIENTED_EDGE('',*,*,#4292,.F.);
#5677=ORIENTED_EDGE('',*,*,#4293,.T.);
#5678=ORIENTED_EDGE('',*,*,#4292,.T.);
#5679=ORIENTED_EDGE('',*,*,#4294,.F.);
#5680=ORIENTED_EDGE('',*,*,#4295,.F.);
#5681=ORIENTED_EDGE('',*,*,#4296,.T.);
#5682=ORIENTED_EDGE('',*,*,#4295,.T.);
#5683=ORIENTED_EDGE('',*,*,#4297,.F.);
#5684=ORIENTED_EDGE('',*,*,#4298,.F.);
#5685=ORIENTED_EDGE('',*,*,#4299,.T.);
#5686=ORIENTED_EDGE('',*,*,#4298,.T.);
#5687=ORIENTED_EDGE('',*,*,#4300,.F.);
#5688=ORIENTED_EDGE('',*,*,#4301,.F.);
#5689=ORIENTED_EDGE('',*,*,#4302,.T.);
#5690=ORIENTED_EDGE('',*,*,#4301,.T.);
#5691=ORIENTED_EDGE('',*,*,#4303,.F.);
#5692=ORIENTED_EDGE('',*,*,#4304,.F.);
#5693=ORIENTED_EDGE('',*,*,#4305,.T.);
#5694=ORIENTED_EDGE('',*,*,#4304,.T.);
#5695=ORIENTED_EDGE('',*,*,#4306,.F.);
#5696=ORIENTED_EDGE('',*,*,#4307,.F.);
#5697=ORIENTED_EDGE('',*,*,#4308,.T.);
#5698=ORIENTED_EDGE('',*,*,#4307,.T.);
#5699=ORIENTED_EDGE('',*,*,#4309,.F.);
#5700=ORIENTED_EDGE('',*,*,#4310,.F.);
#5701=ORIENTED_EDGE('',*,*,#4311,.T.);
#5702=ORIENTED_EDGE('',*,*,#4310,.T.);
#5703=ORIENTED_EDGE('',*,*,#4312,.F.);
#5704=ORIENTED_EDGE('',*,*,#4313,.F.);
#5705=ORIENTED_EDGE('',*,*,#4314,.T.);
#5706=ORIENTED_EDGE('',*,*,#4313,.T.);
#5707=ORIENTED_EDGE('',*,*,#4315,.F.);
#5708=ORIENTED_EDGE('',*,*,#4316,.F.);
#5709=ORIENTED_EDGE('',*,*,#4317,.T.);
#5710=ORIENTED_EDGE('',*,*,#4316,.T.);
#5711=ORIENTED_EDGE('',*,*,#4318,.F.);
#5712=ORIENTED_EDGE('',*,*,#4319,.F.);
#5713=ORIENTED_EDGE('',*,*,#4320,.T.);
#5714=ORIENTED_EDGE('',*,*,#4319,.T.);
#5715=ORIENTED_EDGE('',*,*,#4321,.F.);
#5716=ORIENTED_EDGE('',*,*,#4269,.F.);
#5717=ORIENTED_EDGE('',*,*,#4320,.F.);
#5718=ORIENTED_EDGE('',*,*,#4268,.F.);
#5719=ORIENTED_EDGE('',*,*,#4272,.F.);
#5720=ORIENTED_EDGE('',*,*,#4275,.F.);
#5721=ORIENTED_EDGE('',*,*,#4278,.F.);
#5722=ORIENTED_EDGE('',*,*,#4281,.F.);
#5723=ORIENTED_EDGE('',*,*,#4284,.F.);
#5724=ORIENTED_EDGE('',*,*,#4287,.F.);
#5725=ORIENTED_EDGE('',*,*,#4290,.F.);
#5726=ORIENTED_EDGE('',*,*,#4293,.F.);
#5727=ORIENTED_EDGE('',*,*,#4296,.F.);
#5728=ORIENTED_EDGE('',*,*,#4299,.F.);
#5729=ORIENTED_EDGE('',*,*,#4302,.F.);
#5730=ORIENTED_EDGE('',*,*,#4305,.F.);
#5731=ORIENTED_EDGE('',*,*,#4308,.F.);
#5732=ORIENTED_EDGE('',*,*,#4311,.F.);
#5733=ORIENTED_EDGE('',*,*,#4314,.F.);
#5734=ORIENTED_EDGE('',*,*,#4317,.F.);
#5735=ORIENTED_EDGE('',*,*,#4318,.T.);
#5736=ORIENTED_EDGE('',*,*,#4322,.F.);
#5737=ORIENTED_EDGE('',*,*,#4315,.T.);
#5738=ORIENTED_EDGE('',*,*,#4323,.F.);
#5739=ORIENTED_EDGE('',*,*,#4312,.T.);
#5740=ORIENTED_EDGE('',*,*,#4324,.F.);
#5741=ORIENTED_EDGE('',*,*,#4309,.T.);
#5742=ORIENTED_EDGE('',*,*,#4325,.F.);
#5743=ORIENTED_EDGE('',*,*,#4306,.T.);
#5744=ORIENTED_EDGE('',*,*,#4326,.F.);
#5745=ORIENTED_EDGE('',*,*,#4303,.T.);
#5746=ORIENTED_EDGE('',*,*,#4327,.F.);
#5747=ORIENTED_EDGE('',*,*,#4294,.T.);
#5748=ORIENTED_EDGE('',*,*,#4291,.T.);
#5749=ORIENTED_EDGE('',*,*,#4288,.T.);
#5750=ORIENTED_EDGE('',*,*,#4285,.T.);
#5751=ORIENTED_EDGE('',*,*,#4282,.T.);
#5752=ORIENTED_EDGE('',*,*,#4279,.T.);
#5753=ORIENTED_EDGE('',*,*,#4276,.T.);
#5754=ORIENTED_EDGE('',*,*,#4273,.T.);
#5755=ORIENTED_EDGE('',*,*,#4270,.T.);
#5756=ORIENTED_EDGE('',*,*,#4321,.T.);
#5757=ORIENTED_EDGE('',*,*,#4328,.F.);
#5758=ORIENTED_EDGE('',*,*,#4329,.F.);
#5759=ORIENTED_EDGE('',*,*,#4330,.T.);
#5760=ORIENTED_EDGE('',*,*,#4331,.T.);
#5761=ORIENTED_EDGE('',*,*,#4332,.T.);
#5762=ORIENTED_EDGE('',*,*,#4333,.T.);
#5763=ORIENTED_EDGE('',*,*,#4334,.T.);
#5764=ORIENTED_EDGE('',*,*,#4335,.T.);
#5765=ORIENTED_EDGE('',*,*,#4336,.T.);
#5766=ORIENTED_EDGE('',*,*,#4337,.T.);
#5767=ORIENTED_EDGE('',*,*,#4338,.T.);
#5768=ORIENTED_EDGE('',*,*,#4339,.T.);
#5769=ORIENTED_EDGE('',*,*,#4340,.F.);
#5770=ORIENTED_EDGE('',*,*,#4341,.T.);
#5771=ORIENTED_EDGE('',*,*,#4342,.T.);
#5772=ORIENTED_EDGE('',*,*,#4343,.T.);
#5773=ORIENTED_EDGE('',*,*,#4344,.T.);
#5774=ORIENTED_EDGE('',*,*,#4345,.T.);
#5775=ORIENTED_EDGE('',*,*,#4346,.T.);
#5776=ORIENTED_EDGE('',*,*,#4347,.T.);
#5777=ORIENTED_EDGE('',*,*,#4348,.T.);
#5778=ORIENTED_EDGE('',*,*,#4349,.T.);
#5779=ORIENTED_EDGE('',*,*,#4350,.T.);
#5780=ORIENTED_EDGE('',*,*,#4351,.F.);
#5781=ORIENTED_EDGE('',*,*,#4265,.T.);
#5782=ORIENTED_EDGE('',*,*,#4297,.T.);
#5783=ORIENTED_EDGE('',*,*,#4352,.F.);
#5784=ORIENTED_EDGE('',*,*,#4300,.T.);
#5785=ORIENTED_EDGE('',*,*,#4353,.F.);
#5786=ORIENTED_EDGE('',*,*,#4354,.T.);
#5787=ORIENTED_EDGE('',*,*,#4355,.T.);
#5788=ORIENTED_EDGE('',*,*,#4338,.F.);
#5789=ORIENTED_EDGE('',*,*,#4356,.F.);
#5790=ORIENTED_EDGE('',*,*,#4357,.T.);
#5791=ORIENTED_EDGE('',*,*,#4356,.T.);
#5792=ORIENTED_EDGE('',*,*,#4337,.F.);
#5793=ORIENTED_EDGE('',*,*,#4358,.F.);
#5794=ORIENTED_EDGE('',*,*,#4359,.T.);
#5795=ORIENTED_EDGE('',*,*,#4358,.T.);
#5796=ORIENTED_EDGE('',*,*,#4336,.F.);
#5797=ORIENTED_EDGE('',*,*,#4360,.F.);
#5798=ORIENTED_EDGE('',*,*,#4361,.T.);
#5799=ORIENTED_EDGE('',*,*,#4360,.T.);
#5800=ORIENTED_EDGE('',*,*,#4335,.F.);
#5801=ORIENTED_EDGE('',*,*,#4362,.F.);
#5802=ORIENTED_EDGE('',*,*,#4363,.T.);
#5803=ORIENTED_EDGE('',*,*,#4362,.T.);
#5804=ORIENTED_EDGE('',*,*,#4334,.F.);
#5805=ORIENTED_EDGE('',*,*,#4364,.F.);
#5806=ORIENTED_EDGE('',*,*,#4365,.T.);
#5807=ORIENTED_EDGE('',*,*,#4364,.T.);
#5808=ORIENTED_EDGE('',*,*,#4333,.F.);
#5809=ORIENTED_EDGE('',*,*,#4366,.F.);
#5810=ORIENTED_EDGE('',*,*,#4367,.T.);
#5811=ORIENTED_EDGE('',*,*,#4366,.T.);
#5812=ORIENTED_EDGE('',*,*,#4332,.F.);
#5813=ORIENTED_EDGE('',*,*,#4368,.F.);
#5814=ORIENTED_EDGE('',*,*,#4369,.T.);
#5815=ORIENTED_EDGE('',*,*,#4368,.T.);
#5816=ORIENTED_EDGE('',*,*,#4331,.F.);
#5817=ORIENTED_EDGE('',*,*,#4370,.F.);
#5818=ORIENTED_EDGE('',*,*,#4371,.T.);
#5819=ORIENTED_EDGE('',*,*,#4370,.T.);
#5820=ORIENTED_EDGE('',*,*,#4330,.F.);
#5821=ORIENTED_EDGE('',*,*,#4372,.F.);
#5822=ORIENTED_EDGE('',*,*,#4373,.T.);
#5823=ORIENTED_EDGE('',*,*,#4372,.T.);
#5824=ORIENTED_EDGE('',*,*,#4374,.F.);
#5825=ORIENTED_EDGE('',*,*,#4375,.F.);
#5826=ORIENTED_EDGE('',*,*,#4376,.T.);
#5827=ORIENTED_EDGE('',*,*,#4375,.T.);
#5828=ORIENTED_EDGE('',*,*,#4377,.F.);
#5829=ORIENTED_EDGE('',*,*,#4378,.F.);
#5830=ORIENTED_EDGE('',*,*,#4379,.T.);
#5831=ORIENTED_EDGE('',*,*,#4378,.T.);
#5832=ORIENTED_EDGE('',*,*,#4380,.F.);
#5833=ORIENTED_EDGE('',*,*,#4381,.F.);
#5834=ORIENTED_EDGE('',*,*,#4382,.T.);
#5835=ORIENTED_EDGE('',*,*,#4381,.T.);
#5836=ORIENTED_EDGE('',*,*,#4383,.F.);
#5837=ORIENTED_EDGE('',*,*,#4384,.F.);
#5838=ORIENTED_EDGE('',*,*,#4385,.T.);
#5839=ORIENTED_EDGE('',*,*,#4384,.T.);
#5840=ORIENTED_EDGE('',*,*,#4386,.F.);
#5841=ORIENTED_EDGE('',*,*,#4387,.F.);
#5842=ORIENTED_EDGE('',*,*,#4388,.T.);
#5843=ORIENTED_EDGE('',*,*,#4387,.T.);
#5844=ORIENTED_EDGE('',*,*,#4389,.F.);
#5845=ORIENTED_EDGE('',*,*,#4390,.F.);
#5846=ORIENTED_EDGE('',*,*,#4391,.T.);
#5847=ORIENTED_EDGE('',*,*,#4390,.T.);
#5848=ORIENTED_EDGE('',*,*,#4392,.F.);
#5849=ORIENTED_EDGE('',*,*,#4393,.F.);
#5850=ORIENTED_EDGE('',*,*,#4394,.T.);
#5851=ORIENTED_EDGE('',*,*,#4393,.T.);
#5852=ORIENTED_EDGE('',*,*,#4395,.F.);
#5853=ORIENTED_EDGE('',*,*,#4396,.F.);
#5854=ORIENTED_EDGE('',*,*,#4397,.T.);
#5855=ORIENTED_EDGE('',*,*,#4396,.T.);
#5856=ORIENTED_EDGE('',*,*,#4339,.F.);
#5857=ORIENTED_EDGE('',*,*,#4355,.F.);
#5858=ORIENTED_EDGE('',*,*,#4397,.F.);
#5859=ORIENTED_EDGE('',*,*,#4354,.F.);
#5860=ORIENTED_EDGE('',*,*,#4357,.F.);
#5861=ORIENTED_EDGE('',*,*,#4359,.F.);
#5862=ORIENTED_EDGE('',*,*,#4361,.F.);
#5863=ORIENTED_EDGE('',*,*,#4363,.F.);
#5864=ORIENTED_EDGE('',*,*,#4365,.F.);
#5865=ORIENTED_EDGE('',*,*,#4367,.F.);
#5866=ORIENTED_EDGE('',*,*,#4369,.F.);
#5867=ORIENTED_EDGE('',*,*,#4371,.F.);
#5868=ORIENTED_EDGE('',*,*,#4373,.F.);
#5869=ORIENTED_EDGE('',*,*,#4376,.F.);
#5870=ORIENTED_EDGE('',*,*,#4379,.F.);
#5871=ORIENTED_EDGE('',*,*,#4382,.F.);
#5872=ORIENTED_EDGE('',*,*,#4385,.F.);
#5873=ORIENTED_EDGE('',*,*,#4388,.F.);
#5874=ORIENTED_EDGE('',*,*,#4391,.F.);
#5875=ORIENTED_EDGE('',*,*,#4394,.F.);
#5876=ORIENTED_EDGE('',*,*,#4395,.T.);
#5877=ORIENTED_EDGE('',*,*,#4398,.F.);
#5878=ORIENTED_EDGE('',*,*,#4392,.T.);
#5879=ORIENTED_EDGE('',*,*,#4399,.F.);
#5880=ORIENTED_EDGE('',*,*,#4389,.T.);
#5881=ORIENTED_EDGE('',*,*,#4400,.F.);
#5882=ORIENTED_EDGE('',*,*,#4386,.T.);
#5883=ORIENTED_EDGE('',*,*,#4401,.F.);
#5884=ORIENTED_EDGE('',*,*,#4383,.T.);
#5885=ORIENTED_EDGE('',*,*,#4402,.F.);
#5886=ORIENTED_EDGE('',*,*,#4380,.T.);
#5887=ORIENTED_EDGE('',*,*,#4403,.F.);
#5888=ORIENTED_EDGE('',*,*,#4374,.T.);
#5889=ORIENTED_EDGE('',*,*,#4404,.F.);
#5890=ORIENTED_EDGE('',*,*,#4377,.T.);
#5891=ORIENTED_EDGE('',*,*,#4405,.F.);
#5892=ORIENTED_EDGE('',*,*,#4406,.T.);
#5893=ORIENTED_EDGE('',*,*,#4407,.T.);
#5894=ORIENTED_EDGE('',*,*,#4349,.F.);
#5895=ORIENTED_EDGE('',*,*,#4408,.F.);
#5896=ORIENTED_EDGE('',*,*,#4409,.T.);
#5897=ORIENTED_EDGE('',*,*,#4408,.T.);
#5898=ORIENTED_EDGE('',*,*,#4348,.F.);
#5899=ORIENTED_EDGE('',*,*,#4410,.F.);
#5900=ORIENTED_EDGE('',*,*,#4411,.T.);
#5901=ORIENTED_EDGE('',*,*,#4410,.T.);
#5902=ORIENTED_EDGE('',*,*,#4347,.F.);
#5903=ORIENTED_EDGE('',*,*,#4412,.F.);
#5904=ORIENTED_EDGE('',*,*,#4413,.T.);
#5905=ORIENTED_EDGE('',*,*,#4412,.T.);
#5906=ORIENTED_EDGE('',*,*,#4346,.F.);
#5907=ORIENTED_EDGE('',*,*,#4414,.F.);
#5908=ORIENTED_EDGE('',*,*,#4415,.T.);
#5909=ORIENTED_EDGE('',*,*,#4414,.T.);
#5910=ORIENTED_EDGE('',*,*,#4345,.F.);
#5911=ORIENTED_EDGE('',*,*,#4416,.F.);
#5912=ORIENTED_EDGE('',*,*,#4417,.T.);
#5913=ORIENTED_EDGE('',*,*,#4416,.T.);
#5914=ORIENTED_EDGE('',*,*,#4344,.F.);
#5915=ORIENTED_EDGE('',*,*,#4418,.F.);
#5916=ORIENTED_EDGE('',*,*,#4419,.T.);
#5917=ORIENTED_EDGE('',*,*,#4418,.T.);
#5918=ORIENTED_EDGE('',*,*,#4343,.F.);
#5919=ORIENTED_EDGE('',*,*,#4420,.F.);
#5920=ORIENTED_EDGE('',*,*,#4421,.T.);
#5921=ORIENTED_EDGE('',*,*,#4420,.T.);
#5922=ORIENTED_EDGE('',*,*,#4342,.F.);
#5923=ORIENTED_EDGE('',*,*,#4422,.F.);
#5924=ORIENTED_EDGE('',*,*,#4423,.T.);
#5925=ORIENTED_EDGE('',*,*,#4422,.T.);
#5926=ORIENTED_EDGE('',*,*,#4341,.F.);
#5927=ORIENTED_EDGE('',*,*,#4424,.F.);
#5928=ORIENTED_EDGE('',*,*,#4425,.T.);
#5929=ORIENTED_EDGE('',*,*,#4424,.T.);
#5930=ORIENTED_EDGE('',*,*,#4426,.F.);
#5931=ORIENTED_EDGE('',*,*,#4427,.F.);
#5932=ORIENTED_EDGE('',*,*,#4428,.T.);
#5933=ORIENTED_EDGE('',*,*,#4427,.T.);
#5934=ORIENTED_EDGE('',*,*,#4429,.F.);
#5935=ORIENTED_EDGE('',*,*,#4430,.F.);
#5936=ORIENTED_EDGE('',*,*,#4431,.T.);
#5937=ORIENTED_EDGE('',*,*,#4430,.T.);
#5938=ORIENTED_EDGE('',*,*,#4432,.F.);
#5939=ORIENTED_EDGE('',*,*,#4433,.F.);
#5940=ORIENTED_EDGE('',*,*,#4434,.T.);
#5941=ORIENTED_EDGE('',*,*,#4433,.T.);
#5942=ORIENTED_EDGE('',*,*,#4435,.F.);
#5943=ORIENTED_EDGE('',*,*,#4436,.F.);
#5944=ORIENTED_EDGE('',*,*,#4437,.T.);
#5945=ORIENTED_EDGE('',*,*,#4436,.T.);
#5946=ORIENTED_EDGE('',*,*,#4438,.F.);
#5947=ORIENTED_EDGE('',*,*,#4439,.F.);
#5948=ORIENTED_EDGE('',*,*,#4440,.T.);
#5949=ORIENTED_EDGE('',*,*,#4439,.T.);
#5950=ORIENTED_EDGE('',*,*,#4441,.F.);
#5951=ORIENTED_EDGE('',*,*,#4442,.F.);
#5952=ORIENTED_EDGE('',*,*,#4443,.T.);
#5953=ORIENTED_EDGE('',*,*,#4442,.T.);
#5954=ORIENTED_EDGE('',*,*,#4444,.F.);
#5955=ORIENTED_EDGE('',*,*,#4445,.F.);
#5956=ORIENTED_EDGE('',*,*,#4446,.T.);
#5957=ORIENTED_EDGE('',*,*,#4445,.T.);
#5958=ORIENTED_EDGE('',*,*,#4447,.F.);
#5959=ORIENTED_EDGE('',*,*,#4448,.F.);
#5960=ORIENTED_EDGE('',*,*,#4449,.T.);
#5961=ORIENTED_EDGE('',*,*,#4448,.T.);
#5962=ORIENTED_EDGE('',*,*,#4350,.F.);
#5963=ORIENTED_EDGE('',*,*,#4407,.F.);
#5964=ORIENTED_EDGE('',*,*,#4449,.F.);
#5965=ORIENTED_EDGE('',*,*,#4406,.F.);
#5966=ORIENTED_EDGE('',*,*,#4409,.F.);
#5967=ORIENTED_EDGE('',*,*,#4411,.F.);
#5968=ORIENTED_EDGE('',*,*,#4413,.F.);
#5969=ORIENTED_EDGE('',*,*,#4415,.F.);
#5970=ORIENTED_EDGE('',*,*,#4417,.F.);
#5971=ORIENTED_EDGE('',*,*,#4419,.F.);
#5972=ORIENTED_EDGE('',*,*,#4421,.F.);
#5973=ORIENTED_EDGE('',*,*,#4423,.F.);
#5974=ORIENTED_EDGE('',*,*,#4425,.F.);
#5975=ORIENTED_EDGE('',*,*,#4428,.F.);
#5976=ORIENTED_EDGE('',*,*,#4431,.F.);
#5977=ORIENTED_EDGE('',*,*,#4434,.F.);
#5978=ORIENTED_EDGE('',*,*,#4437,.F.);
#5979=ORIENTED_EDGE('',*,*,#4440,.F.);
#5980=ORIENTED_EDGE('',*,*,#4443,.F.);
#5981=ORIENTED_EDGE('',*,*,#4446,.F.);
#5982=ORIENTED_EDGE('',*,*,#4447,.T.);
#5983=ORIENTED_EDGE('',*,*,#4450,.F.);
#5984=ORIENTED_EDGE('',*,*,#4444,.T.);
#5985=ORIENTED_EDGE('',*,*,#4451,.F.);
#5986=ORIENTED_EDGE('',*,*,#4441,.T.);
#5987=ORIENTED_EDGE('',*,*,#4452,.F.);
#5988=ORIENTED_EDGE('',*,*,#4438,.T.);
#5989=ORIENTED_EDGE('',*,*,#4453,.F.);
#5990=ORIENTED_EDGE('',*,*,#4435,.T.);
#5991=ORIENTED_EDGE('',*,*,#4454,.F.);
#5992=ORIENTED_EDGE('',*,*,#4432,.T.);
#5993=ORIENTED_EDGE('',*,*,#4455,.F.);
#5994=ORIENTED_EDGE('',*,*,#4426,.T.);
#5995=ORIENTED_EDGE('',*,*,#4456,.F.);
#5996=ORIENTED_EDGE('',*,*,#4429,.T.);
#5997=ORIENTED_EDGE('',*,*,#4457,.F.);
#5998=ORIENTED_EDGE('',*,*,#4458,.F.);
#5999=ORIENTED_EDGE('',*,*,#4459,.T.);
#6000=ORIENTED_EDGE('',*,*,#4328,.T.);
#6001=ORIENTED_EDGE('',*,*,#4322,.T.);
#6002=ORIENTED_EDGE('',*,*,#4323,.T.);
#6003=ORIENTED_EDGE('',*,*,#4324,.T.);
#6004=ORIENTED_EDGE('',*,*,#4325,.T.);
#6005=ORIENTED_EDGE('',*,*,#4326,.T.);
#6006=ORIENTED_EDGE('',*,*,#4327,.T.);
#6007=ORIENTED_EDGE('',*,*,#4353,.T.);
#6008=ORIENTED_EDGE('',*,*,#4352,.T.);
#6009=ORIENTED_EDGE('',*,*,#4351,.T.);
#6010=ORIENTED_EDGE('',*,*,#4450,.T.);
#6011=ORIENTED_EDGE('',*,*,#4451,.T.);
#6012=ORIENTED_EDGE('',*,*,#4452,.T.);
#6013=ORIENTED_EDGE('',*,*,#4453,.T.);
#6014=ORIENTED_EDGE('',*,*,#4454,.T.);
#6015=ORIENTED_EDGE('',*,*,#4455,.T.);
#6016=ORIENTED_EDGE('',*,*,#4457,.T.);
#6017=ORIENTED_EDGE('',*,*,#4456,.T.);
#6018=ORIENTED_EDGE('',*,*,#4340,.T.);
#6019=ORIENTED_EDGE('',*,*,#4398,.T.);
#6020=ORIENTED_EDGE('',*,*,#4399,.T.);
#6021=ORIENTED_EDGE('',*,*,#4400,.T.);
#6022=ORIENTED_EDGE('',*,*,#4401,.T.);
#6023=ORIENTED_EDGE('',*,*,#4402,.T.);
#6024=ORIENTED_EDGE('',*,*,#4403,.T.);
#6025=ORIENTED_EDGE('',*,*,#4405,.T.);
#6026=ORIENTED_EDGE('',*,*,#4404,.T.);
#6027=ORIENTED_EDGE('',*,*,#4329,.T.);
#6028=ORIENTED_EDGE('',*,*,#4459,.F.);
#6029=ORIENTED_EDGE('',*,*,#4263,.T.);
#6030=ORIENTED_EDGE('',*,*,#4264,.T.);
#6031=ORIENTED_EDGE('',*,*,#4458,.T.);
#6032=ORIENTED_EDGE('',*,*,#4267,.T.);
#6934=CYLINDRICAL_SURFACE('',#7736,0.21);
#6935=CYLINDRICAL_SURFACE('',#7737,0.6);
#6936=CYLINDRICAL_SURFACE('',#7850,1.37);
#7109=ADVANCED_FACE('',(#718),#6934,.F.);
#7110=ADVANCED_FACE('',(#719,#189),#6935,.F.);
#7111=ADVANCED_FACE('',(#720),#327,.T.);
#7112=ADVANCED_FACE('',(#721),#328,.T.);
#7113=ADVANCED_FACE('',(#722),#329,.T.);
#7114=ADVANCED_FACE('',(#723),#330,.T.);
#7115=ADVANCED_FACE('',(#724),#331,.T.);
#7116=ADVANCED_FACE('',(#725),#332,.T.);
#7117=ADVANCED_FACE('',(#726),#333,.T.);
#7118=ADVANCED_FACE('',(#727),#334,.T.);
#7119=ADVANCED_FACE('',(#728),#335,.T.);
#7120=ADVANCED_FACE('',(#729),#336,.T.);
#7121=ADVANCED_FACE('',(#730),#337,.T.);
#7122=ADVANCED_FACE('',(#731),#338,.T.);
#7123=ADVANCED_FACE('',(#732),#339,.T.);
#7124=ADVANCED_FACE('',(#733),#340,.T.);
#7125=ADVANCED_FACE('',(#734),#341,.T.);
#7126=ADVANCED_FACE('',(#735),#342,.T.);
#7127=ADVANCED_FACE('',(#736),#343,.T.);
#7128=ADVANCED_FACE('',(#737),#344,.T.);
#7129=ADVANCED_FACE('',(#738),#345,.F.);
#7130=ADVANCED_FACE('',(#739),#346,.F.);
#7131=ADVANCED_FACE('',(#740),#347,.F.);
#7132=ADVANCED_FACE('',(#741),#348,.F.);
#7133=ADVANCED_FACE('',(#742),#349,.F.);
#7134=ADVANCED_FACE('',(#743),#350,.F.);
#7135=ADVANCED_FACE('',(#744),#351,.F.);
#7136=ADVANCED_FACE('',(#745,#190),#352,.F.);
#7137=ADVANCED_FACE('',(#746),#353,.F.);
#7138=ADVANCED_FACE('',(#747),#354,.F.);
#7139=ADVANCED_FACE('',(#748),#355,.T.);
#7140=ADVANCED_FACE('',(#749),#356,.T.);
#7141=ADVANCED_FACE('',(#750),#357,.T.);
#7142=ADVANCED_FACE('',(#751),#358,.T.);
#7143=ADVANCED_FACE('',(#752),#359,.T.);
#7144=ADVANCED_FACE('',(#753),#360,.T.);
#7145=ADVANCED_FACE('',(#754),#361,.T.);
#7146=ADVANCED_FACE('',(#755),#362,.T.);
#7147=ADVANCED_FACE('',(#756),#363,.T.);
#7148=ADVANCED_FACE('',(#757),#364,.T.);
#7149=ADVANCED_FACE('',(#758),#365,.T.);
#7150=ADVANCED_FACE('',(#759),#366,.T.);
#7151=ADVANCED_FACE('',(#760),#367,.T.);
#7152=ADVANCED_FACE('',(#761),#368,.T.);
#7153=ADVANCED_FACE('',(#762),#369,.T.);
#7154=ADVANCED_FACE('',(#763),#370,.T.);
#7155=ADVANCED_FACE('',(#764),#371,.T.);
#7156=ADVANCED_FACE('',(#765),#372,.T.);
#7157=ADVANCED_FACE('',(#766),#373,.F.);
#7158=ADVANCED_FACE('',(#767),#374,.F.);
#7159=ADVANCED_FACE('',(#768),#375,.F.);
#7160=ADVANCED_FACE('',(#769),#376,.F.);
#7161=ADVANCED_FACE('',(#770),#377,.F.);
#7162=ADVANCED_FACE('',(#771),#378,.F.);
#7163=ADVANCED_FACE('',(#772),#379,.F.);
#7164=ADVANCED_FACE('',(#773),#380,.F.);
#7165=ADVANCED_FACE('',(#774),#381,.F.);
#7166=ADVANCED_FACE('',(#775),#382,.T.);
#7167=ADVANCED_FACE('',(#776),#383,.T.);
#7168=ADVANCED_FACE('',(#777),#384,.T.);
#7169=ADVANCED_FACE('',(#778),#385,.T.);
#7170=ADVANCED_FACE('',(#779),#386,.T.);
#7171=ADVANCED_FACE('',(#780),#387,.T.);
#7172=ADVANCED_FACE('',(#781),#388,.T.);
#7173=ADVANCED_FACE('',(#782),#389,.T.);
#7174=ADVANCED_FACE('',(#783),#390,.T.);
#7175=ADVANCED_FACE('',(#784),#391,.T.);
#7176=ADVANCED_FACE('',(#785),#392,.T.);
#7177=ADVANCED_FACE('',(#786),#393,.T.);
#7178=ADVANCED_FACE('',(#787),#394,.T.);
#7179=ADVANCED_FACE('',(#788),#395,.T.);
#7180=ADVANCED_FACE('',(#789),#396,.T.);
#7181=ADVANCED_FACE('',(#790),#397,.T.);
#7182=ADVANCED_FACE('',(#791),#398,.T.);
#7183=ADVANCED_FACE('',(#792),#399,.T.);
#7184=ADVANCED_FACE('',(#793),#400,.F.);
#7185=ADVANCED_FACE('',(#794),#401,.F.);
#7186=ADVANCED_FACE('',(#795),#402,.F.);
#7187=ADVANCED_FACE('',(#796),#403,.F.);
#7188=ADVANCED_FACE('',(#797),#404,.F.);
#7189=ADVANCED_FACE('',(#798),#405,.F.);
#7190=ADVANCED_FACE('',(#799),#406,.F.);
#7191=ADVANCED_FACE('',(#800),#407,.F.);
#7192=ADVANCED_FACE('',(#801),#408,.F.);
#7193=ADVANCED_FACE('',(#802,#191),#6936,.T.);
#7194=ADVANCED_FACE('',(#803,#192),#409,.T.);
#7357=CLOSED_SHELL('',(#7109,#7110,#7111,#7112,#7113,#7114,#7115,#7116,
#7117,#7118,#7119,#7120,#7121,#7122,#7123,#7124,#7125,#7126,#7127,#7128,
#7129,#7130,#7131,#7132,#7133,#7134,#7135,#7136,#7137,#7138,#7139,#7140,
#7141,#7142,#7143,#7144,#7145,#7146,#7147,#7148,#7149,#7150,#7151,#7152,
#7153,#7154,#7155,#7156,#7157,#7158,#7159,#7160,#7161,#7162,#7163,#7164,
#7165,#7166,#7167,#7168,#7169,#7170,#7171,#7172,#7173,#7174,#7175,#7176,
#7177,#7178,#7179,#7180,#7181,#7182,#7183,#7184,#7185,#7186,#7187,#7188,
#7189,#7190,#7191,#7192,#7193,#7194));
#7735=AXIS2_PLACEMENT_3D('',#10939,#8834,#8835);
#7736=AXIS2_PLACEMENT_3D('',#10940,#8836,#8837);
#7737=AXIS2_PLACEMENT_3D('',#11018,#8839,#8840);
#7738=AXIS2_PLACEMENT_3D('',#11020,#8841,#8842);
#7739=AXIS2_PLACEMENT_3D('',#11023,#8844,#8845);
#7740=AXIS2_PLACEMENT_3D('',#11024,#8846,#8847);
#7741=AXIS2_PLACEMENT_3D('',#11033,#8852,#8853);
#7742=AXIS2_PLACEMENT_3D('',#11039,#8857,#8858);
#7743=AXIS2_PLACEMENT_3D('',#11045,#8862,#8863);
#7744=AXIS2_PLACEMENT_3D('',#11051,#8867,#8868);
#7745=AXIS2_PLACEMENT_3D('',#11057,#8872,#8873);
#7746=AXIS2_PLACEMENT_3D('',#11063,#8877,#8878);
#7747=AXIS2_PLACEMENT_3D('',#11069,#8882,#8883);
#7748=AXIS2_PLACEMENT_3D('',#11075,#8887,#8888);
#7749=AXIS2_PLACEMENT_3D('',#11081,#8892,#8893);
#7750=AXIS2_PLACEMENT_3D('',#11087,#8897,#8898);
#7751=AXIS2_PLACEMENT_3D('',#11093,#8902,#8903);
#7752=AXIS2_PLACEMENT_3D('',#11099,#8907,#8908);
#7753=AXIS2_PLACEMENT_3D('',#11105,#8912,#8913);
#7754=AXIS2_PLACEMENT_3D('',#11111,#8917,#8918);
#7755=AXIS2_PLACEMENT_3D('',#11117,#8922,#8923);
#7756=AXIS2_PLACEMENT_3D('',#11123,#8927,#8928);
#7757=AXIS2_PLACEMENT_3D('',#11129,#8932,#8933);
#7758=AXIS2_PLACEMENT_3D('',#11132,#8936,#8937);
#7759=AXIS2_PLACEMENT_3D('',#11133,#8938,#8939);
#7760=AXIS2_PLACEMENT_3D('',#11134,#8940,#8941);
#7761=AXIS2_PLACEMENT_3D('',#11135,#8942,#8943);
#7762=AXIS2_PLACEMENT_3D('',#11136,#8944,#8945);
#7763=AXIS2_PLACEMENT_3D('',#11137,#8946,#8947);
#7764=AXIS2_PLACEMENT_3D('',#11138,#8948,#8949);
#7765=AXIS2_PLACEMENT_3D('',#11139,#8950,#8951);
#7766=AXIS2_PLACEMENT_3D('',#11140,#8952,#8953);
#7767=AXIS2_PLACEMENT_3D('',#11141,#8954,#8955);
#7768=AXIS2_PLACEMENT_3D('',#11142,#8956,#8957);
#7769=AXIS2_PLACEMENT_3D('',#11143,#8958,#8959);
#7770=AXIS2_PLACEMENT_3D('',#11144,#8960,#8961);
#7771=AXIS2_PLACEMENT_3D('',#11145,#8962,#8963);
#7772=AXIS2_PLACEMENT_3D('',#11147,#8964,#8965);
#7773=AXIS2_PLACEMENT_3D('',#11149,#8966,#8967);
#7774=AXIS2_PLACEMENT_3D('',#11171,#8978,#8979);
#7775=AXIS2_PLACEMENT_3D('',#11192,#8990,#8991);
#7776=AXIS2_PLACEMENT_3D('',#11193,#8992,#8993);
#7777=AXIS2_PLACEMENT_3D('',#11194,#8994,#8995);
#7778=AXIS2_PLACEMENT_3D('',#11195,#8996,#8997);
#7779=AXIS2_PLACEMENT_3D('',#11196,#8998,#8999);
#7780=AXIS2_PLACEMENT_3D('',#11197,#9000,#9001);
#7781=AXIS2_PLACEMENT_3D('',#11203,#9005,#9006);
#7782=AXIS2_PLACEMENT_3D('',#11207,#9009,#9010);
#7783=AXIS2_PLACEMENT_3D('',#11211,#9013,#9014);
#7784=AXIS2_PLACEMENT_3D('',#11215,#9017,#9018);
#7785=AXIS2_PLACEMENT_3D('',#11219,#9021,#9022);
#7786=AXIS2_PLACEMENT_3D('',#11223,#9025,#9026);
#7787=AXIS2_PLACEMENT_3D('',#11227,#9029,#9030);
#7788=AXIS2_PLACEMENT_3D('',#11231,#9033,#9034);
#7789=AXIS2_PLACEMENT_3D('',#11235,#9037,#9038);
#7790=AXIS2_PLACEMENT_3D('',#11241,#9042,#9043);
#7791=AXIS2_PLACEMENT_3D('',#11247,#9047,#9048);
#7792=AXIS2_PLACEMENT_3D('',#11253,#9052,#9053);
#7793=AXIS2_PLACEMENT_3D('',#11259,#9057,#9058);
#7794=AXIS2_PLACEMENT_3D('',#11265,#9062,#9063);
#7795=AXIS2_PLACEMENT_3D('',#11271,#9067,#9068);
#7796=AXIS2_PLACEMENT_3D('',#11277,#9072,#9073);
#7797=AXIS2_PLACEMENT_3D('',#11282,#9077,#9078);
#7798=AXIS2_PLACEMENT_3D('',#11284,#9080,#9081);
#7799=AXIS2_PLACEMENT_3D('',#11285,#9082,#9083);
#7800=AXIS2_PLACEMENT_3D('',#11286,#9084,#9085);
#7801=AXIS2_PLACEMENT_3D('',#11287,#9086,#9087);
#7802=AXIS2_PLACEMENT_3D('',#11288,#9088,#9089);
#7803=AXIS2_PLACEMENT_3D('',#11289,#9090,#9091);
#7804=AXIS2_PLACEMENT_3D('',#11290,#9092,#9093);
#7805=AXIS2_PLACEMENT_3D('',#11291,#9094,#9095);
#7806=AXIS2_PLACEMENT_3D('',#11292,#9096,#9097);
#7807=AXIS2_PLACEMENT_3D('',#11293,#9098,#9099);
#7808=AXIS2_PLACEMENT_3D('',#11294,#9100,#9101);
#7809=AXIS2_PLACEMENT_3D('',#11295,#9102,#9103);
#7810=AXIS2_PLACEMENT_3D('',#11296,#9104,#9105);
#7811=AXIS2_PLACEMENT_3D('',#11297,#9106,#9107);
#7812=AXIS2_PLACEMENT_3D('',#11298,#9108,#9109);
#7813=AXIS2_PLACEMENT_3D('',#11299,#9110,#9111);
#7814=AXIS2_PLACEMENT_3D('',#11300,#9112,#9113);
#7815=AXIS2_PLACEMENT_3D('',#11301,#9114,#9115);
#7816=AXIS2_PLACEMENT_3D('',#11307,#9119,#9120);
#7817=AXIS2_PLACEMENT_3D('',#11311,#9123,#9124);
#7818=AXIS2_PLACEMENT_3D('',#11315,#9127,#9128);
#7819=AXIS2_PLACEMENT_3D('',#11319,#9131,#9132);
#7820=AXIS2_PLACEMENT_3D('',#11323,#9135,#9136);
#7821=AXIS2_PLACEMENT_3D('',#11327,#9139,#9140);
#7822=AXIS2_PLACEMENT_3D('',#11331,#9143,#9144);
#7823=AXIS2_PLACEMENT_3D('',#11335,#9147,#9148);
#7824=AXIS2_PLACEMENT_3D('',#11339,#9151,#9152);
#7825=AXIS2_PLACEMENT_3D('',#11345,#9156,#9157);
#7826=AXIS2_PLACEMENT_3D('',#11351,#9161,#9162);
#7827=AXIS2_PLACEMENT_3D('',#11357,#9166,#9167);
#7828=AXIS2_PLACEMENT_3D('',#11363,#9171,#9172);
#7829=AXIS2_PLACEMENT_3D('',#11369,#9176,#9177);
#7830=AXIS2_PLACEMENT_3D('',#11375,#9181,#9182);
#7831=AXIS2_PLACEMENT_3D('',#11381,#9186,#9187);
#7832=AXIS2_PLACEMENT_3D('',#11386,#9191,#9192);
#7833=AXIS2_PLACEMENT_3D('',#11388,#9194,#9195);
#7834=AXIS2_PLACEMENT_3D('',#11389,#9196,#9197);
#7835=AXIS2_PLACEMENT_3D('',#11390,#9198,#9199);
#7836=AXIS2_PLACEMENT_3D('',#11391,#9200,#9201);
#7837=AXIS2_PLACEMENT_3D('',#11392,#9202,#9203);
#7838=AXIS2_PLACEMENT_3D('',#11393,#9204,#9205);
#7839=AXIS2_PLACEMENT_3D('',#11394,#9206,#9207);
#7840=AXIS2_PLACEMENT_3D('',#11395,#9208,#9209);
#7841=AXIS2_PLACEMENT_3D('',#11396,#9210,#9211);
#7842=AXIS2_PLACEMENT_3D('',#11397,#9212,#9213);
#7843=AXIS2_PLACEMENT_3D('',#11398,#9214,#9215);
#7844=AXIS2_PLACEMENT_3D('',#11399,#9216,#9217);
#7845=AXIS2_PLACEMENT_3D('',#11400,#9218,#9219);
#7846=AXIS2_PLACEMENT_3D('',#11401,#9220,#9221);
#7847=AXIS2_PLACEMENT_3D('',#11402,#9222,#9223);
#7848=AXIS2_PLACEMENT_3D('',#11403,#9224,#9225);
#7849=AXIS2_PLACEMENT_3D('',#11404,#9226,#9227);
#7850=AXIS2_PLACEMENT_3D('',#11405,#9228,#9229);
#7851=AXIS2_PLACEMENT_3D('',#11407,#9230,#9231);
#7852=AXIS2_PLACEMENT_3D('',#11409,#9233,#9234);
#8834=DIRECTION('axis',(0.,0.,1.));
#8835=DIRECTION('refdir',(1.,0.,0.));
#8836=DIRECTION('center_axis',(0.866025403784439,0.,0.5));
#8837=DIRECTION('ref_axis',(0.5,0.,-0.866025403784439));
#8838=DIRECTION('',(0.866025403784439,0.,0.5));
#8839=DIRECTION('center_axis',(0.,1.,0.));
#8840=DIRECTION('ref_axis',(0.5,0.,-0.866025403784439));
#8841=DIRECTION('center_axis',(0.,1.,0.));
#8842=DIRECTION('ref_axis',(0.5,0.,-0.866025403784439));
#8843=DIRECTION('',(0.,1.,0.));
#8844=DIRECTION('center_axis',(0.,-1.,0.));
#8845=DIRECTION('ref_axis',(0.5,0.,-0.866025403784439));
#8846=DIRECTION('center_axis',(-0.179016861276632,0.,-0.983846005927078));
#8847=DIRECTION('ref_axis',(-0.983846005927078,0.,0.179016861276632));
#8848=DIRECTION('',(-0.983846005927078,0.,0.179016861276632));
#8849=DIRECTION('',(0.,1.,0.));
#8850=DIRECTION('',(-0.983846005927078,0.,0.179016861276632));
#8851=DIRECTION('',(0.,1.,0.));
#8852=DIRECTION('center_axis',(-0.274588618184931,0.,-0.961561797682962));
#8853=DIRECTION('ref_axis',(-0.961561797682962,0.,0.274588618184931));
#8854=DIRECTION('',(-0.961561797682962,0.,0.274588618184931));
#8855=DIRECTION('',(-0.961561797682962,0.,0.274588618184931));
#8856=DIRECTION('',(0.,1.,0.));
#8857=DIRECTION('center_axis',(-0.367515936594703,0.,-0.930017223684013));
#8858=DIRECTION('ref_axis',(-0.930017223684012,0.,0.367515936594703));
#8859=DIRECTION('',(-0.930017223684012,0.,0.367515936594703));
#8860=DIRECTION('',(-0.930017223684013,0.,0.367515936594703));
#8861=DIRECTION('',(0.,1.,0.));
#8862=DIRECTION('center_axis',(-0.45690387563042,0.,-0.889516075421857));
#8863=DIRECTION('ref_axis',(-0.889516075421857,0.,0.45690387563042));
#8864=DIRECTION('',(-0.889516075421857,0.,0.45690387563042));
#8865=DIRECTION('',(-0.889516075421857,0.,0.45690387563042));
#8866=DIRECTION('',(0.,1.,0.));
#8867=DIRECTION('center_axis',(-0.541891580574751,0.,-0.840448401094438));
#8868=DIRECTION('ref_axis',(-0.840448401094438,0.,0.541891580574751));
#8869=DIRECTION('',(-0.840448401094438,0.,0.541891580574751));
#8870=DIRECTION('',(-0.840448401094438,0.,0.541891580574751));
#8871=DIRECTION('',(0.,1.,0.));
#8872=DIRECTION('center_axis',(-0.621660573370077,0.,-0.783286749228651));
#8873=DIRECTION('ref_axis',(-0.783286749228651,0.,0.621660573370077));
#8874=DIRECTION('',(-0.783286749228651,0.,0.621660573370077));
#8875=DIRECTION('',(-0.783286749228651,0.,0.621660573370077));
#8876=DIRECTION('',(0.,1.,0.));
#8877=DIRECTION('center_axis',(-0.695442635009612,0.,-0.718581617779698));
#8878=DIRECTION('ref_axis',(-0.718581617779698,0.,0.695442635009612));
#8879=DIRECTION('',(-0.718581617779698,0.,0.695442635009612));
#8880=DIRECTION('',(-0.718581617779698,0.,0.695442635009612));
#8881=DIRECTION('',(0.,1.,0.));
#8882=DIRECTION('center_axis',(-0.762527203906388,0.,-0.646956152534857));
#8883=DIRECTION('ref_axis',(-0.646956152534857,0.,0.762527203906388));
#8884=DIRECTION('',(-0.646956152534858,0.,0.762527203906388));
#8885=DIRECTION('',(-0.646956152534857,0.,0.762527203906388));
#8886=DIRECTION('',(0.,1.,0.));
#8887=DIRECTION('center_axis',(0.608761429008721,0.,-0.793353340291235));
#8888=DIRECTION('ref_axis',(-0.793353340291235,0.,-0.608761429008721));
#8889=DIRECTION('',(-0.793353340291235,0.,-0.608761429008721));
#8890=DIRECTION('',(-0.793353340291235,0.,-0.608761429008721));
#8891=DIRECTION('',(0.,1.,0.));
#8892=DIRECTION('center_axis',(0.762527203906388,0.,0.646956152534857));
#8893=DIRECTION('ref_axis',(0.646956152534857,0.,-0.762527203906388));
#8894=DIRECTION('',(0.646956152534857,0.,-0.762527203906388));
#8895=DIRECTION('',(0.646956152534857,0.,-0.762527203906388));
#8896=DIRECTION('',(0.,1.,0.));
#8897=DIRECTION('center_axis',(0.695442635009612,0.,0.718581617779698));
#8898=DIRECTION('ref_axis',(0.718581617779698,0.,-0.695442635009612));
#8899=DIRECTION('',(0.718581617779698,0.,-0.695442635009612));
#8900=DIRECTION('',(0.718581617779698,0.,-0.695442635009612));
#8901=DIRECTION('',(0.,1.,0.));
#8902=DIRECTION('center_axis',(0.621660573370078,0.,0.78328674922865));
#8903=DIRECTION('ref_axis',(0.78328674922865,0.,-0.621660573370078));
#8904=DIRECTION('',(0.78328674922865,0.,-0.621660573370078));
#8905=DIRECTION('',(0.78328674922865,0.,-0.621660573370078));
#8906=DIRECTION('',(0.,1.,0.));
#8907=DIRECTION('center_axis',(0.54189158057475,0.,0.84044840109444));
#8908=DIRECTION('ref_axis',(0.84044840109444,0.,-0.54189158057475));
#8909=DIRECTION('',(0.84044840109444,0.,-0.54189158057475));
#8910=DIRECTION('',(0.84044840109444,0.,-0.54189158057475));
#8911=DIRECTION('',(0.,1.,0.));
#8912=DIRECTION('center_axis',(0.456903875630422,0.,0.889516075421856));
#8913=DIRECTION('ref_axis',(0.889516075421856,0.,-0.456903875630422));
#8914=DIRECTION('',(0.889516075421856,0.,-0.456903875630422));
#8915=DIRECTION('',(0.889516075421856,0.,-0.456903875630422));
#8916=DIRECTION('',(0.,1.,0.));
#8917=DIRECTION('center_axis',(0.367515936594702,0.,0.930017223684013));
#8918=DIRECTION('ref_axis',(0.930017223684013,0.,-0.367515936594702));
#8919=DIRECTION('',(0.930017223684013,0.,-0.367515936594702));
#8920=DIRECTION('',(0.930017223684013,0.,-0.367515936594702));
#8921=DIRECTION('',(0.,1.,0.));
#8922=DIRECTION('center_axis',(0.274588618184931,0.,0.961561797682962));
#8923=DIRECTION('ref_axis',(0.961561797682962,0.,-0.274588618184931));
#8924=DIRECTION('',(0.961561797682962,0.,-0.274588618184931));
#8925=DIRECTION('',(0.961561797682962,0.,-0.274588618184931));
#8926=DIRECTION('',(0.,1.,0.));
#8927=DIRECTION('center_axis',(0.179016861276631,0.,0.983846005927078));
#8928=DIRECTION('ref_axis',(0.983846005927078,0.,-0.179016861276631));
#8929=DIRECTION('',(0.983846005927078,0.,-0.179016861276631));
#8930=DIRECTION('',(0.983846005927078,0.,-0.179016861276631));
#8931=DIRECTION('',(0.,1.,0.));
#8932=DIRECTION('center_axis',(-0.99144486137381,0.,0.130526192220051));
#8933=DIRECTION('ref_axis',(0.130526192220051,0.,0.99144486137381));
#8934=DIRECTION('',(0.130526192220051,0.,0.99144486137381));
#8935=DIRECTION('',(0.130526192220051,0.,0.99144486137381));
#8936=DIRECTION('center_axis',(0.,1.,0.));
#8937=DIRECTION('ref_axis',(0.499999999999999,0.,0.866025403784439));
#8938=DIRECTION('center_axis',(0.,1.,0.));
#8939=DIRECTION('ref_axis',(0.5,0.,-0.866025403784439));
#8940=DIRECTION('center_axis',(0.,1.,0.));
#8941=DIRECTION('ref_axis',(0.5,0.,-0.866025403784438));
#8942=DIRECTION('center_axis',(0.,1.,0.));
#8943=DIRECTION('ref_axis',(0.5,0.,-0.866025403784439));
#8944=DIRECTION('center_axis',(0.,1.,0.));
#8945=DIRECTION('ref_axis',(0.5,0.,-0.866025403784438));
#8946=DIRECTION('center_axis',(0.,1.,0.));
#8947=DIRECTION('ref_axis',(0.5,0.,-0.866025403784439));
#8948=DIRECTION('center_axis',(0.,1.,0.));
#8949=DIRECTION('ref_axis',(0.5,0.,-0.866025403784438));
#8950=DIRECTION('center_axis',(0.,1.,0.));
#8951=DIRECTION('ref_axis',(0.5,0.,-0.866025403784439));
#8952=DIRECTION('center_axis',(0.,1.,0.));
#8953=DIRECTION('ref_axis',(0.5,0.,-0.866025403784438));
#8954=DIRECTION('center_axis',(0.,1.,0.));
#8955=DIRECTION('ref_axis',(0.5,0.,-0.866025403784439));
#8956=DIRECTION('center_axis',(0.,1.,0.));
#8957=DIRECTION('ref_axis',(0.5,0.,-0.866025403784438));
#8958=DIRECTION('center_axis',(0.,1.,0.));
#8959=DIRECTION('ref_axis',(0.5,0.,-0.866025403784439));
#8960=DIRECTION('center_axis',(0.,1.,0.));
#8961=DIRECTION('ref_axis',(0.5,0.,-0.866025403784438));
#8962=DIRECTION('center_axis',(0.,1.,0.));
#8963=DIRECTION('ref_axis',(0.5,0.,-0.866025403784439));
#8964=DIRECTION('center_axis',(0.,1.,0.));
#8965=DIRECTION('ref_axis',(0.5,0.,-0.866025403784438));
#8966=DIRECTION('center_axis',(0.,1.,0.));
#8967=DIRECTION('ref_axis',(0.5,0.,-0.866025403784438));
#8968=DIRECTION('',(0.923879532511287,0.,-0.38268343236509));
#8969=DIRECTION('',(-0.33688985339222,0.,-0.941544065183021));
#8970=DIRECTION('',(-0.242980179903264,0.,-0.970031253194544));
#8971=DIRECTION('',(-0.146730474455362,0.,-0.989176509964781));
#8972=DIRECTION('',(-0.0490676743274178,0.,-0.998795456205172));
#8973=DIRECTION('',(0.0490676743274185,0.,-0.998795456205172));
#8974=DIRECTION('',(0.146730474455362,0.,-0.989176509964781));
#8975=DIRECTION('',(0.242980179903265,0.,-0.970031253194544));
#8976=DIRECTION('',(0.336889853392221,0.,-0.941544065183021));
#8977=DIRECTION('',(-0.923879532511287,0.,-0.38268343236509));
#8978=DIRECTION('center_axis',(0.,1.,0.));
#8979=DIRECTION('ref_axis',(0.5,0.,-0.866025403784438));
#8980=DIRECTION('',(-0.130526192220052,0.,0.99144486137381));
#8981=DIRECTION('',(0.983846005927078,0.,0.179016861276632));
#8982=DIRECTION('',(0.961561797682962,0.,0.274588618184932));
#8983=DIRECTION('',(0.930017223684012,0.,0.367515936594704));
#8984=DIRECTION('',(0.889516075421856,0.,0.456903875630421));
#8985=DIRECTION('',(0.840448401094438,0.,0.541891580574752));
#8986=DIRECTION('',(0.78328674922865,0.,0.621660573370078));
#8987=DIRECTION('',(0.718581617779698,0.,0.695442635009612));
#8988=DIRECTION('',(0.646956152534857,0.,0.762527203906389));
#8989=DIRECTION('',(0.793353340291235,0.,-0.60876142900872));
#8990=DIRECTION('center_axis',(0.,1.,0.));
#8991=DIRECTION('ref_axis',(0.5,0.,-0.866025403784438));
#8992=DIRECTION('center_axis',(0.,1.,0.));
#8993=DIRECTION('ref_axis',(0.5,0.,-0.866025403784439));
#8994=DIRECTION('center_axis',(0.,1.,0.));
#8995=DIRECTION('ref_axis',(0.5,0.,-0.866025403784438));
#8996=DIRECTION('center_axis',(0.,1.,0.));
#8997=DIRECTION('ref_axis',(0.5,0.,-0.866025403784439));
#8998=DIRECTION('center_axis',(0.,1.,0.));
#8999=DIRECTION('ref_axis',(0.5,0.,-0.866025403784438));
#9000=DIRECTION('center_axis',(0.941544065183021,0.,0.336889853392221));
#9001=DIRECTION('ref_axis',(0.336889853392221,0.,-0.941544065183021));
#9002=DIRECTION('',(0.336889853392221,0.,-0.941544065183021));
#9003=DIRECTION('',(0.,1.,0.));
#9004=DIRECTION('',(0.,1.,0.));
#9005=DIRECTION('center_axis',(0.970031253194544,0.,0.242980179903265));
#9006=DIRECTION('ref_axis',(0.242980179903265,0.,-0.970031253194544));
#9007=DIRECTION('',(0.242980179903265,0.,-0.970031253194544));
#9008=DIRECTION('',(0.,1.,0.));
#9009=DIRECTION('center_axis',(0.989176509964781,0.,0.146730474455362));
#9010=DIRECTION('ref_axis',(0.146730474455362,0.,-0.989176509964781));
#9011=DIRECTION('',(0.146730474455362,0.,-0.989176509964781));
#9012=DIRECTION('',(0.,1.,0.));
#9013=DIRECTION('center_axis',(0.998795456205172,0.,0.0490676743274185));
#9014=DIRECTION('ref_axis',(0.0490676743274185,0.,-0.998795456205172));
#9015=DIRECTION('',(0.0490676743274185,0.,-0.998795456205172));
#9016=DIRECTION('',(0.,1.,0.));
#9017=DIRECTION('center_axis',(0.998795456205172,0.,-0.0490676743274178));
#9018=DIRECTION('ref_axis',(-0.0490676743274178,0.,-0.998795456205172));
#9019=DIRECTION('',(-0.0490676743274178,0.,-0.998795456205172));
#9020=DIRECTION('',(0.,1.,0.));
#9021=DIRECTION('center_axis',(0.989176509964781,0.,-0.146730474455361));
#9022=DIRECTION('ref_axis',(-0.146730474455361,0.,-0.989176509964781));
#9023=DIRECTION('',(-0.146730474455361,0.,-0.989176509964781));
#9024=DIRECTION('',(0.,1.,0.));
#9025=DIRECTION('center_axis',(0.970031253194544,0.,-0.242980179903264));
#9026=DIRECTION('ref_axis',(-0.242980179903264,0.,-0.970031253194544));
#9027=DIRECTION('',(-0.242980179903264,0.,-0.970031253194544));
#9028=DIRECTION('',(0.,1.,0.));
#9029=DIRECTION('center_axis',(0.941544065183021,0.,-0.33688985339222));
#9030=DIRECTION('ref_axis',(-0.33688985339222,0.,-0.941544065183021));
#9031=DIRECTION('',(-0.33688985339222,0.,-0.941544065183021));
#9032=DIRECTION('',(0.,1.,0.));
#9033=DIRECTION('center_axis',(0.38268343236509,0.,0.923879532511287));
#9034=DIRECTION('ref_axis',(0.923879532511287,0.,-0.38268343236509));
#9035=DIRECTION('',(0.923879532511287,0.,-0.38268343236509));
#9036=DIRECTION('',(0.,1.,0.));
#9037=DIRECTION('center_axis',(-0.941544065183021,0.,0.336889853392221));
#9038=DIRECTION('ref_axis',(0.336889853392221,0.,0.941544065183021));
#9039=DIRECTION('',(0.336889853392221,0.,0.941544065183021));
#9040=DIRECTION('',(0.336889853392221,0.,0.941544065183021));
#9041=DIRECTION('',(0.,1.,0.));
#9042=DIRECTION('center_axis',(-0.970031253194544,0.,0.242980179903264));
#9043=DIRECTION('ref_axis',(0.242980179903264,0.,0.970031253194544));
#9044=DIRECTION('',(0.242980179903264,0.,0.970031253194544));
#9045=DIRECTION('',(0.242980179903264,0.,0.970031253194544));
#9046=DIRECTION('',(0.,1.,0.));
#9047=DIRECTION('center_axis',(-0.989176509964781,0.,0.146730474455362));
#9048=DIRECTION('ref_axis',(0.146730474455362,0.,0.989176509964781));
#9049=DIRECTION('',(0.146730474455362,0.,0.989176509964781));
#9050=DIRECTION('',(0.146730474455362,0.,0.989176509964781));
#9051=DIRECTION('',(0.,1.,0.));
#9052=DIRECTION('center_axis',(-0.998795456205173,0.,0.0490676743274157));
#9053=DIRECTION('ref_axis',(0.0490676743274157,0.,0.998795456205173));
#9054=DIRECTION('',(0.0490676743274157,0.,0.998795456205173));
#9055=DIRECTION('',(0.0490676743274157,0.,0.998795456205173));
#9056=DIRECTION('',(0.,1.,0.));
#9057=DIRECTION('center_axis',(-0.998795456205173,0.,-0.0490676743274162));
#9058=DIRECTION('ref_axis',(-0.0490676743274162,0.,0.998795456205173));
#9059=DIRECTION('',(-0.0490676743274162,0.,0.998795456205173));
#9060=DIRECTION('',(-0.0490676743274162,0.,0.998795456205173));
#9061=DIRECTION('',(0.,1.,0.));
#9062=DIRECTION('center_axis',(-0.989176509964781,0.,-0.146730474455363));
#9063=DIRECTION('ref_axis',(-0.146730474455363,0.,0.989176509964781));
#9064=DIRECTION('',(-0.146730474455363,0.,0.989176509964781));
#9065=DIRECTION('',(-0.146730474455363,0.,0.989176509964781));
#9066=DIRECTION('',(0.,1.,0.));
#9067=DIRECTION('center_axis',(-0.970031253194544,0.,-0.242980179903265));
#9068=DIRECTION('ref_axis',(-0.242980179903265,0.,0.970031253194544));
#9069=DIRECTION('',(-0.242980179903265,0.,0.970031253194544));
#9070=DIRECTION('',(-0.242980179903265,0.,0.970031253194544));
#9071=DIRECTION('',(0.,1.,0.));
#9072=DIRECTION('center_axis',(-0.94154406518302,0.,-0.336889853392221));
#9073=DIRECTION('ref_axis',(-0.336889853392221,0.,0.94154406518302));
#9074=DIRECTION('',(-0.336889853392221,0.,0.94154406518302));
#9075=DIRECTION('',(-0.336889853392221,0.,0.94154406518302));
#9076=DIRECTION('',(0.,1.,0.));
#9077=DIRECTION('center_axis',(0.38268343236509,0.,-0.923879532511287));
#9078=DIRECTION('ref_axis',(-0.923879532511287,0.,-0.38268343236509));
#9079=DIRECTION('',(-0.923879532511287,0.,-0.38268343236509));
#9080=DIRECTION('center_axis',(0.,1.,0.));
#9081=DIRECTION('ref_axis',(-1.,0.,-3.33066907387547E-16));
#9082=DIRECTION('center_axis',(0.,1.,0.));
#9083=DIRECTION('ref_axis',(0.5,0.,-0.866025403784439));
#9084=DIRECTION('center_axis',(0.,1.,0.));
#9085=DIRECTION('ref_axis',(0.5,0.,-0.866025403784438));
#9086=DIRECTION('center_axis',(0.,1.,0.));
#9087=DIRECTION('ref_axis',(0.5,0.,-0.866025403784439));
#9088=DIRECTION('center_axis',(0.,1.,0.));
#9089=DIRECTION('ref_axis',(0.5,0.,-0.866025403784438));
#9090=DIRECTION('center_axis',(0.,1.,0.));
#9091=DIRECTION('ref_axis',(0.5,0.,-0.866025403784439));
#9092=DIRECTION('center_axis',(0.,1.,0.));
#9093=DIRECTION('ref_axis',(0.5,0.,-0.866025403784438));
#9094=DIRECTION('center_axis',(0.,1.,0.));
#9095=DIRECTION('ref_axis',(0.5,0.,-0.866025403784439));
#9096=DIRECTION('center_axis',(0.,1.,0.));
#9097=DIRECTION('ref_axis',(0.5,0.,-0.866025403784438));
#9098=DIRECTION('center_axis',(0.,1.,0.));
#9099=DIRECTION('ref_axis',(0.5,0.,-0.866025403784439));
#9100=DIRECTION('center_axis',(0.,1.,0.));
#9101=DIRECTION('ref_axis',(0.5,0.,-0.866025403784438));
#9102=DIRECTION('center_axis',(0.,1.,0.));
#9103=DIRECTION('ref_axis',(0.5,0.,-0.866025403784439));
#9104=DIRECTION('center_axis',(0.,1.,0.));
#9105=DIRECTION('ref_axis',(0.5,0.,-0.866025403784438));
#9106=DIRECTION('center_axis',(0.,1.,0.));
#9107=DIRECTION('ref_axis',(0.5,0.,-0.866025403784439));
#9108=DIRECTION('center_axis',(0.,1.,0.));
#9109=DIRECTION('ref_axis',(0.5,0.,-0.866025403784438));
#9110=DIRECTION('center_axis',(0.,1.,0.));
#9111=DIRECTION('ref_axis',(0.5,0.,-0.866025403784439));
#9112=DIRECTION('center_axis',(0.,1.,0.));
#9113=DIRECTION('ref_axis',(0.5,0.,-0.866025403784438));
#9114=DIRECTION('center_axis',(-0.762527203906389,0.,0.646956152534857));
#9115=DIRECTION('ref_axis',(0.646956152534857,0.,0.762527203906389));
#9116=DIRECTION('',(0.646956152534857,0.,0.762527203906389));
#9117=DIRECTION('',(0.,1.,0.));
#9118=DIRECTION('',(0.,1.,0.));
#9119=DIRECTION('center_axis',(-0.695442635009612,0.,0.718581617779698));
#9120=DIRECTION('ref_axis',(0.718581617779698,0.,0.695442635009612));
#9121=DIRECTION('',(0.718581617779698,0.,0.695442635009612));
#9122=DIRECTION('',(0.,1.,0.));
#9123=DIRECTION('center_axis',(-0.621660573370078,0.,0.78328674922865));
#9124=DIRECTION('ref_axis',(0.78328674922865,0.,0.621660573370078));
#9125=DIRECTION('',(0.78328674922865,0.,0.621660573370078));
#9126=DIRECTION('',(0.,1.,0.));
#9127=DIRECTION('center_axis',(-0.541891580574752,0.,0.840448401094438));
#9128=DIRECTION('ref_axis',(0.840448401094438,0.,0.541891580574752));
#9129=DIRECTION('',(0.840448401094438,0.,0.541891580574752));
#9130=DIRECTION('',(0.,1.,0.));
#9131=DIRECTION('center_axis',(-0.456903875630421,0.,0.889516075421856));
#9132=DIRECTION('ref_axis',(0.889516075421856,0.,0.456903875630421));
#9133=DIRECTION('',(0.889516075421856,0.,0.456903875630421));
#9134=DIRECTION('',(0.,1.,0.));
#9135=DIRECTION('center_axis',(-0.367515936594704,0.,0.930017223684012));
#9136=DIRECTION('ref_axis',(0.930017223684012,0.,0.367515936594704));
#9137=DIRECTION('',(0.930017223684012,0.,0.367515936594704));
#9138=DIRECTION('',(0.,1.,0.));
#9139=DIRECTION('center_axis',(-0.274588618184932,0.,0.961561797682962));
#9140=DIRECTION('ref_axis',(0.961561797682962,0.,0.274588618184932));
#9141=DIRECTION('',(0.961561797682962,0.,0.274588618184932));
#9142=DIRECTION('',(0.,1.,0.));
#9143=DIRECTION('center_axis',(-0.179016861276632,0.,0.983846005927078));
#9144=DIRECTION('ref_axis',(0.983846005927078,0.,0.179016861276632));
#9145=DIRECTION('',(0.983846005927077,0.,0.179016861276632));
#9146=DIRECTION('',(0.,1.,0.));
#9147=DIRECTION('center_axis',(-0.99144486137381,0.,-0.130526192220052));
#9148=DIRECTION('ref_axis',(-0.130526192220052,0.,0.99144486137381));
#9149=DIRECTION('',(-0.130526192220052,0.,0.99144486137381));
#9150=DIRECTION('',(0.,1.,0.));
#9151=DIRECTION('center_axis',(0.179016861276632,0.,-0.983846005927078));
#9152=DIRECTION('ref_axis',(-0.983846005927078,0.,-0.179016861276632));
#9153=DIRECTION('',(-0.983846005927078,0.,-0.179016861276632));
#9154=DIRECTION('',(-0.983846005927078,0.,-0.179016861276632));
#9155=DIRECTION('',(0.,1.,0.));
#9156=DIRECTION('center_axis',(0.274588618184932,0.,-0.961561797682962));
#9157=DIRECTION('ref_axis',(-0.961561797682962,0.,-0.274588618184932));
#9158=DIRECTION('',(-0.961561797682962,0.,-0.274588618184932));
#9159=DIRECTION('',(-0.961561797682962,0.,-0.274588618184932));
#9160=DIRECTION('',(0.,1.,0.));
#9161=DIRECTION('center_axis',(0.367515936594703,0.,-0.930017223684013));
#9162=DIRECTION('ref_axis',(-0.930017223684013,0.,-0.367515936594703));
#9163=DIRECTION('',(-0.930017223684013,0.,-0.367515936594703));
#9164=DIRECTION('',(-0.930017223684013,0.,-0.367515936594703));
#9165=DIRECTION('',(0.,1.,0.));
#9166=DIRECTION('center_axis',(0.456903875630423,0.,-0.889516075421855));
#9167=DIRECTION('ref_axis',(-0.889516075421855,0.,-0.456903875630423));
#9168=DIRECTION('',(-0.889516075421855,0.,-0.456903875630423));
#9169=DIRECTION('',(-0.889516075421855,0.,-0.456903875630423));
#9170=DIRECTION('',(0.,1.,0.));
#9171=DIRECTION('center_axis',(0.54189158057475,0.,-0.840448401094439));
#9172=DIRECTION('ref_axis',(-0.840448401094439,0.,-0.54189158057475));
#9173=DIRECTION('',(-0.840448401094439,0.,-0.54189158057475));
#9174=DIRECTION('',(-0.840448401094439,0.,-0.54189158057475));
#9175=DIRECTION('',(0.,1.,0.));
#9176=DIRECTION('center_axis',(0.621660573370078,0.,-0.78328674922865));
#9177=DIRECTION('ref_axis',(-0.78328674922865,0.,-0.621660573370078));
#9178=DIRECTION('',(-0.78328674922865,0.,-0.621660573370078));
#9179=DIRECTION('',(-0.78328674922865,0.,-0.621660573370078));
#9180=DIRECTION('',(0.,1.,0.));
#9181=DIRECTION('center_axis',(0.695442635009612,0.,-0.718581617779698));
#9182=DIRECTION('ref_axis',(-0.718581617779698,0.,-0.695442635009612));
#9183=DIRECTION('',(-0.718581617779698,0.,-0.695442635009612));
#9184=DIRECTION('',(-0.718581617779698,0.,-0.695442635009612));
#9185=DIRECTION('',(0.,1.,0.));
#9186=DIRECTION('center_axis',(0.762527203906389,0.,-0.646956152534857));
#9187=DIRECTION('ref_axis',(-0.646956152534857,0.,-0.762527203906389));
#9188=DIRECTION('',(-0.646956152534857,0.,-0.762527203906389));
#9189=DIRECTION('',(-0.646956152534857,0.,-0.762527203906389));
#9190=DIRECTION('',(0.,1.,0.));
#9191=DIRECTION('center_axis',(0.60876142900872,0.,0.793353340291235));
#9192=DIRECTION('ref_axis',(0.793353340291235,0.,-0.60876142900872));
#9193=DIRECTION('',(0.793353340291235,0.,-0.60876142900872));
#9194=DIRECTION('center_axis',(0.,1.,0.));
#9195=DIRECTION('ref_axis',(0.5,0.,-0.866025403784439));
#9196=DIRECTION('center_axis',(0.,1.,0.));
#9197=DIRECTION('ref_axis',(0.5,0.,-0.866025403784439));
#9198=DIRECTION('center_axis',(0.,1.,0.));
#9199=DIRECTION('ref_axis',(0.5,0.,-0.866025403784438));
#9200=DIRECTION('center_axis',(0.,1.,0.));
#9201=DIRECTION('ref_axis',(0.5,0.,-0.866025403784439));
#9202=DIRECTION('center_axis',(0.,1.,0.));
#9203=DIRECTION('ref_axis',(0.5,0.,-0.866025403784438));
#9204=DIRECTION('center_axis',(0.,1.,0.));
#9205=DIRECTION('ref_axis',(0.5,0.,-0.866025403784439));
#9206=DIRECTION('center_axis',(0.,1.,0.));
#9207=DIRECTION('ref_axis',(0.5,0.,-0.866025403784438));
#9208=DIRECTION('center_axis',(0.,1.,0.));
#9209=DIRECTION('ref_axis',(0.5,0.,-0.866025403784439));
#9210=DIRECTION('center_axis',(0.,1.,0.));
#9211=DIRECTION('ref_axis',(0.5,0.,-0.866025403784438));
#9212=DIRECTION('center_axis',(0.,1.,0.));
#9213=DIRECTION('ref_axis',(0.5,0.,-0.866025403784439));
#9214=DIRECTION('center_axis',(0.,1.,0.));
#9215=DIRECTION('ref_axis',(0.5,0.,-0.866025403784438));
#9216=DIRECTION('center_axis',(0.,1.,0.));
#9217=DIRECTION('ref_axis',(0.5,0.,-0.866025403784439));
#9218=DIRECTION('center_axis',(0.,1.,0.));
#9219=DIRECTION('ref_axis',(0.5,0.,-0.866025403784438));
#9220=DIRECTION('center_axis',(0.,1.,0.));
#9221=DIRECTION('ref_axis',(0.5,0.,-0.866025403784439));
#9222=DIRECTION('center_axis',(0.,1.,0.));
#9223=DIRECTION('ref_axis',(0.5,0.,-0.866025403784438));
#9224=DIRECTION('center_axis',(0.,1.,0.));
#9225=DIRECTION('ref_axis',(0.5,0.,-0.866025403784439));
#9226=DIRECTION('center_axis',(0.,1.,0.));
#9227=DIRECTION('ref_axis',(0.5,0.,-0.866025403784438));
#9228=DIRECTION('center_axis',(0.,1.,0.));
#9229=DIRECTION('ref_axis',(0.5,0.,-0.866025403784438));
#9230=DIRECTION('center_axis',(0.,1.,0.));
#9231=DIRECTION('ref_axis',(0.5,0.,-0.866025403784438));
#9232=DIRECTION('',(0.,-1.,0.));
#9233=DIRECTION('center_axis',(0.,1.,0.));
#9234=DIRECTION('ref_axis',(0.5,0.,-0.866025403784439));
#10939=CARTESIAN_POINT('',(0.,0.,0.));
#10940=CARTESIAN_POINT('Origin',(0.,1.525,0.));
#10941=CARTESIAN_POINT('',(0.591749422187638,1.525,0.0991595751331958));
#10942=CARTESIAN_POINT('',(0.381749422187638,1.525,0.46289024472266));
#10943=CARTESIAN_POINT('Ctrl Pts',(0.591749422187639,1.525,0.0991595751331958));
#10944=CARTESIAN_POINT('Ctrl Pts',(0.591749422187639,1.55162128248078,0.0991595751331958));
#10945=CARTESIAN_POINT('Ctrl Pts',(0.590876440724725,1.5798448972882,0.104852434209432));
#10946=CARTESIAN_POINT('Ctrl Pts',(0.586484941382362,1.63150713274392,0.127139324098885));
#10947=CARTESIAN_POINT('Ctrl Pts',(0.582861172497722,1.65496807125954,0.143660692707601));
#10948=CARTESIAN_POINT('Ctrl Pts',(0.572535383770674,1.69200621178927,0.180467056616695));
#10949=CARTESIAN_POINT('Ctrl Pts',(0.565117205136936,1.70813412776081,0.203279332063799));
#10950=CARTESIAN_POINT('Ctrl Pts',(0.545350992210601,1.72963697075952,0.251539733807139));
#10951=CARTESIAN_POINT('Ctrl Pts',(0.532918292013224,1.735,0.276958441950268));
#10952=CARTESIAN_POINT('Ctrl Pts',(0.506312192528102,1.735,0.323041558049732));
#10953=CARTESIAN_POINT('Ctrl Pts',(0.490515295643458,1.72963697075952,0.346517946329861));
#10954=CARTESIAN_POINT('Ctrl Pts',(0.45860366820005,1.70813412776081,0.387766189732349));
#10955=CARTESIAN_POINT('Ctrl Pts',(0.442556747461599,1.69200621178927,0.40559665860253));
#10956=CARTESIAN_POINT('Ctrl Pts',(0.415844395658913,1.65496807125954,0.43294223590881));
#10957=CARTESIAN_POINT('Ctrl Pts',(0.403348355180798,1.63150713274392,0.44434119612471));
#10958=CARTESIAN_POINT('Ctrl Pts',(0.386243092036367,1.5798448972882,0.459287791060626));
#10959=CARTESIAN_POINT('Ctrl Pts',(0.381749422187638,1.55162128248078,0.46289024472266));
#10960=CARTESIAN_POINT('Ctrl Pts',(0.381749422187638,1.525,0.46289024472266));
#10961=CARTESIAN_POINT('Ctrl Pts',(0.381749422187638,1.525,0.46289024472266));
#10962=CARTESIAN_POINT('Ctrl Pts',(0.381749422187638,1.49837871751922,0.46289024472266));
#10963=CARTESIAN_POINT('Ctrl Pts',(0.386243092036367,1.4701551027118,0.459287791060626));
#10964=CARTESIAN_POINT('Ctrl Pts',(0.403348355180798,1.41849286725608,0.44434119612471));
#10965=CARTESIAN_POINT('Ctrl Pts',(0.415844395658914,1.39503192874046,0.43294223590881));
#10966=CARTESIAN_POINT('Ctrl Pts',(0.442556747461599,1.35799378821073,0.40559665860253));
#10967=CARTESIAN_POINT('Ctrl Pts',(0.45860366820005,1.34186587223919,0.387766189732349));
#10968=CARTESIAN_POINT('Ctrl Pts',(0.490515295643458,1.32036302924048,0.346517946329861));
#10969=CARTESIAN_POINT('Ctrl Pts',(0.506312192528102,1.315,0.323041558049732));
#10970=CARTESIAN_POINT('Ctrl Pts',(0.532918292013224,1.315,0.276958441950268));
#10971=CARTESIAN_POINT('Ctrl Pts',(0.545350992210601,1.32036302924048,0.251539733807139));
#10972=CARTESIAN_POINT('Ctrl Pts',(0.565117205136936,1.34186587223919,0.203279332063799));
#10973=CARTESIAN_POINT('Ctrl Pts',(0.572535383770674,1.35799378821073,0.180467056616695));
#10974=CARTESIAN_POINT('Ctrl Pts',(0.582861172497722,1.39503192874046,0.143660692707601));
#10975=CARTESIAN_POINT('Ctrl Pts',(0.586484941382362,1.41849286725608,0.127139324098885));
#10976=CARTESIAN_POINT('Ctrl Pts',(0.590876440724725,1.47015510271179,0.104852434209432));
#10977=CARTESIAN_POINT('Ctrl Pts',(0.591749422187638,1.49837871751922,0.0991595751331958));
#10978=CARTESIAN_POINT('Ctrl Pts',(0.591749422187638,1.525,0.0991595751331958));
#10979=CARTESIAN_POINT('',(1.06743336697656,1.525,0.85877005482555));
#10980=CARTESIAN_POINT('',(-0.105,1.525,0.181865334794732));
#10981=CARTESIAN_POINT('',(1.27743336697656,1.525,0.495039385236086));
#10982=CARTESIAN_POINT('Ctrl Pts',(1.27743336697656,1.525,0.495039385236086));
#10983=CARTESIAN_POINT('Ctrl Pts',(1.27743336697656,1.49858689919462,0.495039385236086));
#10984=CARTESIAN_POINT('Ctrl Pts',(1.27552837579046,1.47044219200607,0.500044675653854));
#10985=CARTESIAN_POINT('Ctrl Pts',(1.26746274883014,1.41871515620915,0.520149492189153));
#10986=CARTESIAN_POINT('Ctrl Pts',(1.26126362373573,1.39512919832077,0.535224213312019));
#10987=CARTESIAN_POINT('Ctrl Pts',(1.24615878616438,1.35788630799087,0.56950781678886));
#10988=CARTESIAN_POINT('Ctrl Pts',(1.23623425750631,1.34173137598416,0.591012782176279));
#10989=CARTESIAN_POINT('Ctrl Pts',(1.213004701181,1.32028707843824,0.6373310309511));
#10990=CARTESIAN_POINT('Ctrl Pts',(1.19966110223798,1.315,0.662126019059738));
#10991=CARTESIAN_POINT('Ctrl Pts',(1.17324850413138,1.315,0.707873980940262));
#10992=CARTESIAN_POINT('Ctrl Pts',(1.15844721401428,1.32028707843824,0.731827370657151));
#10993=CARTESIAN_POINT('Ctrl Pts',(1.12994921207913,1.34173137598416,0.775103880940915));
#10994=CARTESIAN_POINT('Ctrl Pts',(1.11628763007516,1.35788630799087,0.794451257573106));
#10995=CARTESIAN_POINT('Ctrl Pts',(1.09414957731662,1.39512919832077,0.824674232368354));
#10996=CARTESIAN_POINT('Ctrl Pts',(1.08419404841645,1.41871515620915,0.837580192742778));
#10997=CARTESIAN_POINT('Ctrl Pts',(1.07081558003862,1.47044219200607,0.854617638855513));
#10998=CARTESIAN_POINT('Ctrl Pts',(1.06743336697656,1.49858689919462,0.85877005482555));
#10999=CARTESIAN_POINT('Ctrl Pts',(1.06743336697656,1.525,0.85877005482555));
#11000=CARTESIAN_POINT('Ctrl Pts',(1.06743336697656,1.525,0.85877005482555));
#11001=CARTESIAN_POINT('Ctrl Pts',(1.06743336697656,1.55141310080538,0.85877005482555));
#11002=CARTESIAN_POINT('Ctrl Pts',(1.07081558003862,1.57955780799393,0.854617638855513));
#11003=CARTESIAN_POINT('Ctrl Pts',(1.08419404841645,1.63128484379085,0.837580192742778));
#11004=CARTESIAN_POINT('Ctrl Pts',(1.09414957731662,1.65487080167923,0.824674232368354));
#11005=CARTESIAN_POINT('Ctrl Pts',(1.11628763007516,1.69211369200913,0.794451257573106));
#11006=CARTESIAN_POINT('Ctrl Pts',(1.12994921207913,1.70826862401584,0.775103880940915));
#11007=CARTESIAN_POINT('Ctrl Pts',(1.15844721401428,1.72971292156176,0.731827370657151));
#11008=CARTESIAN_POINT('Ctrl Pts',(1.17324850413138,1.735,0.707873980940262));
#11009=CARTESIAN_POINT('Ctrl Pts',(1.19966110223798,1.735,0.662126019059738));
#11010=CARTESIAN_POINT('Ctrl Pts',(1.213004701181,1.72971292156176,0.6373310309511));
#11011=CARTESIAN_POINT('Ctrl Pts',(1.23623425750631,1.70826862401584,0.591012782176279));
#11012=CARTESIAN_POINT('Ctrl Pts',(1.24615878616438,1.69211369200913,0.569507816788861));
#11013=CARTESIAN_POINT('Ctrl Pts',(1.26126362373573,1.65487080167923,0.535224213312019));
#11014=CARTESIAN_POINT('Ctrl Pts',(1.26746274883014,1.63128484379085,0.520149492189153));
#11015=CARTESIAN_POINT('Ctrl Pts',(1.27552837579046,1.57955780799392,0.500044675653854));
#11016=CARTESIAN_POINT('Ctrl Pts',(1.27743336697656,1.55141310080538,0.495039385236086));
#11017=CARTESIAN_POINT('Ctrl Pts',(1.27743336697656,1.525,0.495039385236086));
#11018=CARTESIAN_POINT('Origin',(0.,0.,0.));
#11019=CARTESIAN_POINT('',(-0.3,1.,0.519615242270663));
#11020=CARTESIAN_POINT('Origin',(0.,1.,0.));
#11021=CARTESIAN_POINT('',(-0.3,2.05,0.519615242270663));
#11022=CARTESIAN_POINT('',(-0.3,0.,0.519615242270663));
#11023=CARTESIAN_POINT('Origin',(0.,2.05,0.));
#11024=CARTESIAN_POINT('Origin',(0.181661010427498,0.4,0.779101583421867));
#11025=CARTESIAN_POINT('',(0.181661010427498,0.4,0.779101583421867));
#11026=CARTESIAN_POINT('',(0.104420953776041,0.4,0.793155889099048));
#11027=CARTESIAN_POINT('',(0.181661010427498,0.4,0.779101583421867));
#11028=CARTESIAN_POINT('',(0.104420953776041,1.,0.793155889099048));
#11029=CARTESIAN_POINT('',(0.104420953776041,0.4,0.793155889099048));
#11030=CARTESIAN_POINT('',(0.181661010427498,1.,0.779101583421867));
#11031=CARTESIAN_POINT('',(0.162350996264633,1.,0.782615159841162));
#11032=CARTESIAN_POINT('',(0.181661010427498,0.4,0.779101583421867));
#11033=CARTESIAN_POINT('Origin',(0.257151572242529,0.4,0.757544103596085));
#11034=CARTESIAN_POINT('',(0.257151572242529,0.4,0.757544103596085));
#11035=CARTESIAN_POINT('',(0.257151572242529,0.4,0.757544103596085));
#11036=CARTESIAN_POINT('',(0.257151572242529,1.,0.757544103596085));
#11037=CARTESIAN_POINT('',(0.238278931788771,1.,0.76293347355253));
#11038=CARTESIAN_POINT('',(0.257151572242529,0.4,0.757544103596085));
#11039=CARTESIAN_POINT('Origin',(0.330165623843515,0.4,0.728691059936941));
#11040=CARTESIAN_POINT('',(0.330165623843515,0.4,0.728691059936941));
#11041=CARTESIAN_POINT('',(0.330165623843515,0.4,0.728691059936941));
#11042=CARTESIAN_POINT('',(0.330165623843515,1.,0.728691059936941));
#11043=CARTESIAN_POINT('',(0.311912110943269,1.,0.735904320851727));
#11044=CARTESIAN_POINT('',(0.330165623843515,0.4,0.728691059936941));
#11045=CARTESIAN_POINT('Origin',(0.4,0.4,0.692820323027551));
#11046=CARTESIAN_POINT('',(0.4,0.4,0.692820323027551));
#11047=CARTESIAN_POINT('',(0.4,0.4,0.692820323027551));
#11048=CARTESIAN_POINT('',(0.4,1.,0.692820323027551));
#11049=CARTESIAN_POINT('',(0.382541405960878,1.,0.701788007254899));
#11050=CARTESIAN_POINT('',(0.4,0.4,0.692820323027551));
#11051=CARTESIAN_POINT('Origin',(0.465982157494241,0.4,0.650277347673292));
#11052=CARTESIAN_POINT('',(0.465982157494241,0.4,0.650277347673292));
#11053=CARTESIAN_POINT('',(0.465982157494241,0.4,0.650277347673292));
#11054=CARTESIAN_POINT('',(0.465982157494241,1.,0.650277347673292));
#11055=CARTESIAN_POINT('',(0.449486618120681,1.,0.660913091511857));
#11056=CARTESIAN_POINT('',(0.465982157494241,0.4,0.650277347673292));
#11057=CARTESIAN_POINT('Origin',(0.527476652080055,0.4,0.601471845983182));
#11058=CARTESIAN_POINT('',(0.527476652080055,0.4,0.601471845983182));
#11059=CARTESIAN_POINT('',(0.527476652080055,0.4,0.601471845983182));
#11060=CARTESIAN_POINT('',(0.527476652080055,1.,0.601471845983182));
#11061=CARTESIAN_POINT('',(0.512103028433601,1.,0.61367322140571));
#11062=CARTESIAN_POINT('',(0.527476652080055,0.4,0.601471845983182));
#11063=CARTESIAN_POINT('Origin',(0.583891258158268,0.4,0.546873841618297));
#11064=CARTESIAN_POINT('',(0.583891258158268,0.4,0.546873841618297));
#11065=CARTESIAN_POINT('',(0.583891258158268,0.4,0.546873841618297));
#11066=CARTESIAN_POINT('',(0.583891258158268,1.,0.546873841618297));
#11067=CARTESIAN_POINT('',(0.569787606638715,1.,0.560523342709519));
#11068=CARTESIAN_POINT('',(0.583891258158268,0.4,0.546873841618297));
#11069=CARTESIAN_POINT('Origin',(0.634682672232988,0.4,0.487009143206977));
#11070=CARTESIAN_POINT('',(0.634682672232988,0.4,0.487009143206977));
#11071=CARTESIAN_POINT('',(0.634682672232988,0.4,0.487009143206977));
#11072=CARTESIAN_POINT('',(0.634682672232988,1.,0.487009143206977));
#11073=CARTESIAN_POINT('',(0.621984818714308,1.,0.501975317809807));
#11074=CARTESIAN_POINT('',(0.634682672232988,0.4,0.487009143206977));
#11075=CARTESIAN_POINT('Origin',(1.08689407619899,0.4,0.834003157741948));
#11076=CARTESIAN_POINT('',(1.08689407619899,0.4,0.834003157741948));
#11077=CARTESIAN_POINT('',(1.08689407619899,0.4,0.834003157741948));
#11078=CARTESIAN_POINT('',(1.08689407619899,1.,0.834003157741948));
#11079=CARTESIAN_POINT('',(0.543447038099496,1.,0.417001578870974));
#11080=CARTESIAN_POINT('',(1.08689407619899,0.4,0.834003157741948));
#11081=CARTESIAN_POINT('Origin',(0.999913779596034,0.4,0.936521453771334));
#11082=CARTESIAN_POINT('',(0.999913779596034,0.4,0.936521453771334));
#11083=CARTESIAN_POINT('',(0.999913779596034,0.4,0.936521453771334));
#11084=CARTESIAN_POINT('',(0.999913779596034,1.,0.936521453771334));
#11085=CARTESIAN_POINT('',(1.02165885374677,1.,0.910891879763987));
#11086=CARTESIAN_POINT('',(0.999913779596034,0.4,0.936521453771334));
#11087=CARTESIAN_POINT('Origin',(0.903303766687094,0.4,1.0300205362462));
#11088=CARTESIAN_POINT('',(0.903303766687094,0.4,1.0300205362462));
#11089=CARTESIAN_POINT('',(0.903303766687094,0.4,1.0300205362462));
#11090=CARTESIAN_POINT('',(0.903303766687094,1.,1.0300205362462));
#11091=CARTESIAN_POINT('',(0.927456269914329,1.,1.00664576562748));
#11092=CARTESIAN_POINT('',(0.903303766687094,0.4,1.0300205362462));
#11093=CARTESIAN_POINT('Origin',(0.797994444708888,0.4,1.11359995789051));
#11094=CARTESIAN_POINT('',(0.797994444708888,0.4,1.11359995789051));
#11095=CARTESIAN_POINT('',(0.797994444708888,0.4,1.11359995789051));
#11096=CARTESIAN_POINT('',(0.797994444708888,1.,1.11359995789051));
#11097=CARTESIAN_POINT('',(0.82432177520344,1.,1.09270510247943));
#11098=CARTESIAN_POINT('',(0.797994444708888,0.4,1.11359995789051));
#11099=CARTESIAN_POINT('Origin',(0.684999999999999,0.4,1.18645480318468));
#11100=CARTESIAN_POINT('',(0.684999999999999,0.4,1.18645480318468));
#11101=CARTESIAN_POINT('',(0.684999999999999,0.4,1.18645480318468));
#11102=CARTESIAN_POINT('',(0.684999999999999,1.,1.18645480318468));
#11103=CARTESIAN_POINT('',(0.71324861117722,1.,1.16824109186114));
#11104=CARTESIAN_POINT('',(0.684999999999999,0.4,1.18645480318468));
#11105=CARTESIAN_POINT('Origin',(0.56540863083202,0.4,1.24788344014201));
#11106=CARTESIAN_POINT('',(0.56540863083202,0.4,1.24788344014201));
#11107=CARTESIAN_POINT('',(0.56540863083202,0.4,1.24788344014201));
#11108=CARTESIAN_POINT('',(0.56540863083202,1.,1.24788344014201));
#11109=CARTESIAN_POINT('',(0.595306473124016,1.,1.23252628090268));
#11110=CARTESIAN_POINT('',(0.56540863083202,0.4,1.24788344014201));
#11111=CARTESIAN_POINT('Origin',(0.44037206746533,0.4,1.29729427740829));
#11112=CARTESIAN_POINT('',(0.44037206746533,0.4,1.29729427740829));
#11113=CARTESIAN_POINT('',(0.44037206746533,0.4,1.29729427740829));
#11114=CARTESIAN_POINT('',(0.44037206746533,1.,1.29729427740829));
#11115=CARTESIAN_POINT('',(0.471631208307002,1.,1.28494156809172));
#11116=CARTESIAN_POINT('',(0.44037206746533,0.4,1.29729427740829));
#11117=CARTESIAN_POINT('Origin',(0.311094480357091,0.4,1.33421146160995));
#11118=CARTESIAN_POINT('',(0.311094480357091,0.4,1.33421146160995));
#11119=CARTESIAN_POINT('',(0.311094480357091,0.4,1.33421146160995));
#11120=CARTESIAN_POINT('',(0.311094480357091,1.,1.33421146160995));
#11121=CARTESIAN_POINT('',(0.34341387713415,1.,1.32498216555953));
#11122=CARTESIAN_POINT('',(0.311094480357091,0.4,1.33421146160995));
#11123=CARTESIAN_POINT('Origin',(0.17882088334147,0.4,1.35827946008212));
#11124=CARTESIAN_POINT('',(0.17882088334147,0.4,1.35827946008212));
#11125=CARTESIAN_POINT('',(0.17882088334147,0.4,1.35827946008212));
#11126=CARTESIAN_POINT('',(0.17882088334147,1.,1.35827946008212));
#11127=CARTESIAN_POINT('',(0.211889282595374,1.,1.35226246046408));
#11128=CARTESIAN_POINT('',(0.17882088334147,0.4,1.35827946008212));
#11129=CARTESIAN_POINT('Origin',(0.104420953776041,0.4,0.793155889099048));
#11130=CARTESIAN_POINT('',(0.104420953776041,0.4,0.793155889099048));
#11131=CARTESIAN_POINT('',(0.0522104768880204,1.,0.396577944549524));
#11132=CARTESIAN_POINT('Origin',(0.527275906502257,0.4,0.913268659668847));
#11133=CARTESIAN_POINT('Origin',(0.,1.,0.));
#11134=CARTESIAN_POINT('Origin',(0.,1.,0.));
#11135=CARTESIAN_POINT('Origin',(0.,1.,0.));
#11136=CARTESIAN_POINT('Origin',(0.,1.,0.));
#11137=CARTESIAN_POINT('Origin',(0.,1.,0.));
#11138=CARTESIAN_POINT('Origin',(0.,1.,0.));
#11139=CARTESIAN_POINT('Origin',(0.,1.,0.));
#11140=CARTESIAN_POINT('Origin',(0.,1.,0.));
#11141=CARTESIAN_POINT('Origin',(0.,1.,0.));
#11142=CARTESIAN_POINT('Origin',(0.,1.,0.));
#11143=CARTESIAN_POINT('Origin',(0.,1.,0.));
#11144=CARTESIAN_POINT('Origin',(0.,1.,0.));
#11145=CARTESIAN_POINT('Origin',(0.,1.,0.));
#11146=CARTESIAN_POINT('',(-0.685,1.,1.18645480318468));
#11147=CARTESIAN_POINT('Origin',(0.,1.,0.));
#11148=CARTESIAN_POINT('',(-1.26571495954046,1.,0.524276302340173));
#11149=CARTESIAN_POINT('Origin',(0.,1.,0.));
#11150=CARTESIAN_POINT('',(-0.739103626009029,1.,0.306146745892072));
#11151=CARTESIAN_POINT('',(-0.632857479770231,1.,0.262138151170086));
#11152=CARTESIAN_POINT('',(-0.765552268585767,1.,0.23222774180357));
#11153=CARTESIAN_POINT('',(-0.745715786653214,1.,0.287666994869946));
#11154=CARTESIAN_POINT('',(-0.784628224322584,1.,0.156072257612902));
#11155=CARTESIAN_POINT('',(-0.770321257519971,1.,0.213188870755903));
#11156=CARTESIAN_POINT('',(-0.796147781337758,1.,0.0784137122636482));
#11157=CARTESIAN_POINT('',(-0.787508113576378,1.,0.136657621275589));
#11158=CARTESIAN_POINT('',(-0.8,1.,-2.22044604925031E-16));
#11159=CARTESIAN_POINT('',(-0.797110836003318,1.,0.0588102841977362));
#11160=CARTESIAN_POINT('',(-0.796147781337758,1.,-0.0784137122636487));
#11161=CARTESIAN_POINT('',(-0.799036945334439,1.,-0.0196034280659124));
#11162=CARTESIAN_POINT('',(-0.784628224322584,1.,-0.156072257612903));
#11163=CARTESIAN_POINT('',(-0.793267892083964,1.,-0.0978283486009623));
#11164=CARTESIAN_POINT('',(-0.765552268585767,1.,-0.23222774180357));
#11165=CARTESIAN_POINT('',(-0.77985923538838,1.,-0.17511112866057));
#11166=CARTESIAN_POINT('',(-0.739103626009029,1.,-0.306146745892072));
#11167=CARTESIAN_POINT('',(-0.758940107941583,1.,-0.250707492825696));
#11168=CARTESIAN_POINT('',(-1.26571495954046,1.,-0.524276302340173));
#11169=CARTESIAN_POINT('',(-0.369551813004515,1.,-0.153073372946036));
#11170=CARTESIAN_POINT('',(0.178820883341471,1.,-1.35827946008212));
#11171=CARTESIAN_POINT('Origin',(0.,1.,0.));
#11172=CARTESIAN_POINT('',(0.104420953776041,1.,-0.793155889099048));
#11173=CARTESIAN_POINT('',(0.0894104416707354,1.,-0.67913973004106));
#11174=CARTESIAN_POINT('',(0.181661010427499,1.,-0.779101583421867));
#11175=CARTESIAN_POINT('',(0.123730967938906,1.,-0.789642312679753));
#11176=CARTESIAN_POINT('',(0.257151572242529,1.,-0.757544103596084));
#11177=CARTESIAN_POINT('',(0.200533650881256,1.,-0.773712213465421));
#11178=CARTESIAN_POINT('',(0.330165623843516,1.,-0.728691059936941));
#11179=CARTESIAN_POINT('',(0.275405085142776,1.,-0.750330842681299));
#11180=CARTESIAN_POINT('',(0.4,1.,-0.692820323027551));
#11181=CARTESIAN_POINT('',(0.347624217882637,1.,-0.719723375709593));
#11182=CARTESIAN_POINT('',(0.465982157494242,1.,-0.650277347673292));
#11183=CARTESIAN_POINT('',(0.416495539373561,1.,-0.682184579188986));
#11184=CARTESIAN_POINT('',(0.527476652080055,1.,-0.601471845983182));
#11185=CARTESIAN_POINT('',(0.481355781140695,1.,-0.638075972250765));
#11186=CARTESIAN_POINT('',(0.583891258158269,1.,-0.546873841618297));
#11187=CARTESIAN_POINT('',(0.541580303599609,1.,-0.587822344891961));
#11188=CARTESIAN_POINT('',(0.634682672232988,1.,-0.487009143206976));
#11189=CARTESIAN_POINT('',(0.596589111676949,1.,-0.531907667015467));
#11190=CARTESIAN_POINT('',(1.08689407619899,1.,-0.834003157741947));
#11191=CARTESIAN_POINT('',(0.317341336116494,1.,-0.243504571603488));
#11192=CARTESIAN_POINT('Origin',(0.,1.,0.));
#11193=CARTESIAN_POINT('Origin',(0.,1.,0.));
#11194=CARTESIAN_POINT('Origin',(0.,1.,0.));
#11195=CARTESIAN_POINT('Origin',(0.,1.,0.));
#11196=CARTESIAN_POINT('Origin',(0.,1.,0.));
#11197=CARTESIAN_POINT('Origin',(-0.765552268585767,0.4,-0.23222774180357));
#11198=CARTESIAN_POINT('',(-0.765552268585767,0.4,-0.23222774180357));
#11199=CARTESIAN_POINT('',(-0.739103626009029,0.4,-0.306146745892072));
#11200=CARTESIAN_POINT('',(-0.765552268585767,0.4,-0.23222774180357));
#11201=CARTESIAN_POINT('',(-0.739103626009029,0.4,-0.306146745892072));
#11202=CARTESIAN_POINT('',(-0.765552268585767,0.4,-0.23222774180357));
#11203=CARTESIAN_POINT('Origin',(-0.784628224322584,0.4,-0.156072257612903));
#11204=CARTESIAN_POINT('',(-0.784628224322584,0.4,-0.156072257612903));
#11205=CARTESIAN_POINT('',(-0.784628224322584,0.4,-0.156072257612903));
#11206=CARTESIAN_POINT('',(-0.784628224322584,0.4,-0.156072257612903));
#11207=CARTESIAN_POINT('Origin',(-0.796147781337758,0.4,-0.0784137122636487));
#11208=CARTESIAN_POINT('',(-0.796147781337758,0.4,-0.0784137122636487));
#11209=CARTESIAN_POINT('',(-0.796147781337758,0.4,-0.0784137122636487));
#11210=CARTESIAN_POINT('',(-0.796147781337758,0.4,-0.0784137122636487));
#11211=CARTESIAN_POINT('Origin',(-0.8,0.4,-2.22044604925031E-16));
#11212=CARTESIAN_POINT('',(-0.8,0.4,-2.22044604925031E-16));
#11213=CARTESIAN_POINT('',(-0.8,0.4,-2.22044604925031E-16));
#11214=CARTESIAN_POINT('',(-0.8,0.4,-2.22044604925031E-16));
#11215=CARTESIAN_POINT('Origin',(-0.796147781337758,0.4,0.0784137122636482));
#11216=CARTESIAN_POINT('',(-0.796147781337758,0.4,0.0784137122636482));
#11217=CARTESIAN_POINT('',(-0.796147781337758,0.4,0.0784137122636482));
#11218=CARTESIAN_POINT('',(-0.796147781337758,0.4,0.0784137122636482));
#11219=CARTESIAN_POINT('Origin',(-0.784628224322584,0.4,0.156072257612902));
#11220=CARTESIAN_POINT('',(-0.784628224322584,0.4,0.156072257612902));
#11221=CARTESIAN_POINT('',(-0.784628224322584,0.4,0.156072257612902));
#11222=CARTESIAN_POINT('',(-0.784628224322584,0.4,0.156072257612902));
#11223=CARTESIAN_POINT('Origin',(-0.765552268585767,0.4,0.23222774180357));
#11224=CARTESIAN_POINT('',(-0.765552268585767,0.4,0.23222774180357));
#11225=CARTESIAN_POINT('',(-0.765552268585767,0.4,0.23222774180357));
#11226=CARTESIAN_POINT('',(-0.765552268585767,0.4,0.23222774180357));
#11227=CARTESIAN_POINT('Origin',(-0.739103626009029,0.4,0.306146745892072));
#11228=CARTESIAN_POINT('',(-0.739103626009029,0.4,0.306146745892072));
#11229=CARTESIAN_POINT('',(-0.739103626009029,0.4,0.306146745892072));
#11230=CARTESIAN_POINT('',(-0.739103626009029,0.4,0.306146745892072));
#11231=CARTESIAN_POINT('Origin',(-1.26571495954046,0.4,0.524276302340173));
#11232=CARTESIAN_POINT('',(-1.26571495954046,0.4,0.524276302340173));
#11233=CARTESIAN_POINT('',(-1.26571495954046,0.4,0.524276302340173));
#11234=CARTESIAN_POINT('',(-1.26571495954046,0.4,0.524276302340173));
#11235=CARTESIAN_POINT('Origin',(-1.31100825995313,0.4,0.397690007838613));
#11236=CARTESIAN_POINT('',(-1.31100825995313,0.4,0.397690007838613));
#11237=CARTESIAN_POINT('',(-1.31100825995313,0.4,0.397690007838613));
#11238=CARTESIAN_POINT('',(-1.31100825995313,1.,0.397690007838613));
#11239=CARTESIAN_POINT('',(-1.29968493484996,1.,0.429336581464004));
#11240=CARTESIAN_POINT('',(-1.31100825995313,0.4,0.397690007838613));
#11241=CARTESIAN_POINT('Origin',(-1.34367583415243,0.4,0.267273741162095));
#11242=CARTESIAN_POINT('',(-1.34367583415243,0.4,0.267273741162095));
#11243=CARTESIAN_POINT('',(-1.34367583415243,0.4,0.267273741162095));
#11244=CARTESIAN_POINT('',(-1.34367583415243,1.,0.267273741162095));
#11245=CARTESIAN_POINT('',(-1.3355089406026,1.,0.299877807831225));
#11246=CARTESIAN_POINT('',(-1.34367583415243,0.4,0.267273741162095));
#11247=CARTESIAN_POINT('Origin',(-1.36340307554091,0.4,0.134283482251498));
#11248=CARTESIAN_POINT('',(-1.36340307554091,0.4,0.134283482251498));
#11249=CARTESIAN_POINT('',(-1.36340307554091,0.4,0.134283482251498));
#11250=CARTESIAN_POINT('',(-1.36340307554091,1.,0.134283482251498));
#11251=CARTESIAN_POINT('',(-1.35847126519379,1.,0.167531046979148));
#11252=CARTESIAN_POINT('',(-1.36340307554091,0.4,0.134283482251498));
#11253=CARTESIAN_POINT('Origin',(-1.37,0.4,-3.33066907387547E-16));
#11254=CARTESIAN_POINT('',(-1.37,0.4,-3.33066907387547E-16));
#11255=CARTESIAN_POINT('',(-1.37,0.4,-3.33066907387547E-16));
#11256=CARTESIAN_POINT('',(-1.37,1.,-3.33066907387547E-16));
#11257=CARTESIAN_POINT('',(-1.36835076888523,1.,0.0335708705628729));
#11258=CARTESIAN_POINT('',(-1.37,0.4,-3.33066907387547E-16));
#11259=CARTESIAN_POINT('Origin',(-1.36340307554091,0.4,-0.134283482251498));
#11260=CARTESIAN_POINT('',(-1.36340307554091,0.4,-0.134283482251498));
#11261=CARTESIAN_POINT('',(-1.36340307554091,0.4,-0.134283482251498));
#11262=CARTESIAN_POINT('',(-1.36340307554091,1.,-0.134283482251498));
#11263=CARTESIAN_POINT('',(-1.36505230665568,1.,-0.100712611688622));
#11264=CARTESIAN_POINT('',(-1.36340307554091,0.4,-0.134283482251498));
#11265=CARTESIAN_POINT('Origin',(-1.34367583415243,0.4,-0.267273741162096));
#11266=CARTESIAN_POINT('',(-1.34367583415243,0.4,-0.267273741162096));
#11267=CARTESIAN_POINT('',(-1.34367583415243,0.4,-0.267273741162096));
#11268=CARTESIAN_POINT('',(-1.34367583415243,1.,-0.267273741162096));
#11269=CARTESIAN_POINT('',(-1.34860764449955,1.,-0.234026176434447));
#11270=CARTESIAN_POINT('',(-1.34367583415243,0.4,-0.267273741162096));
#11271=CARTESIAN_POINT('Origin',(-1.31100825995313,0.4,-0.397690007838614));
#11272=CARTESIAN_POINT('',(-1.31100825995313,0.4,-0.397690007838614));
#11273=CARTESIAN_POINT('',(-1.31100825995313,0.4,-0.397690007838614));
#11274=CARTESIAN_POINT('',(-1.31100825995313,1.,-0.397690007838614));
#11275=CARTESIAN_POINT('',(-1.31917515350295,1.,-0.365085941169485));
#11276=CARTESIAN_POINT('',(-1.31100825995313,0.4,-0.397690007838614));
#11277=CARTESIAN_POINT('Origin',(-1.26571495954046,0.4,-0.524276302340173));
#11278=CARTESIAN_POINT('',(-1.26571495954046,0.4,-0.524276302340173));
#11279=CARTESIAN_POINT('',(-1.26571495954046,0.4,-0.524276302340173));
#11280=CARTESIAN_POINT('',(-1.27703828464363,1.,-0.492629728714784));
#11281=CARTESIAN_POINT('',(-1.26571495954046,0.4,-0.524276302340173));
#11282=CARTESIAN_POINT('Origin',(-0.739103626009029,0.4,-0.306146745892072));
#11283=CARTESIAN_POINT('',(-0.739103626009029,0.4,-0.306146745892072));
#11284=CARTESIAN_POINT('Origin',(-1.05455181300451,0.4,-3.33066907387547E-16));
#11285=CARTESIAN_POINT('Origin',(0.,1.,0.));
#11286=CARTESIAN_POINT('Origin',(0.,1.,0.));
#11287=CARTESIAN_POINT('Origin',(0.,1.,0.));
#11288=CARTESIAN_POINT('Origin',(0.,1.,0.));
#11289=CARTESIAN_POINT('Origin',(0.,1.,0.));
#11290=CARTESIAN_POINT('Origin',(0.,1.,0.));
#11291=CARTESIAN_POINT('Origin',(0.,1.,0.));
#11292=CARTESIAN_POINT('Origin',(0.,1.,0.));
#11293=CARTESIAN_POINT('Origin',(0.,1.,0.));
#11294=CARTESIAN_POINT('Origin',(0.,1.,0.));
#11295=CARTESIAN_POINT('Origin',(0.,1.,0.));
#11296=CARTESIAN_POINT('Origin',(0.,1.,0.));
#11297=CARTESIAN_POINT('Origin',(0.,1.,0.));
#11298=CARTESIAN_POINT('Origin',(0.,1.,0.));
#11299=CARTESIAN_POINT('Origin',(0.,1.,0.));
#11300=CARTESIAN_POINT('Origin',(0.,1.,0.));
#11301=CARTESIAN_POINT('Origin',(0.583891258158269,0.4,-0.546873841618297));
#11302=CARTESIAN_POINT('',(0.583891258158269,0.4,-0.546873841618297));
#11303=CARTESIAN_POINT('',(0.634682672232988,0.4,-0.487009143206976));
#11304=CARTESIAN_POINT('',(0.583891258158269,0.4,-0.546873841618297));
#11305=CARTESIAN_POINT('',(0.634682672232988,0.4,-0.487009143206976));
#11306=CARTESIAN_POINT('',(0.583891258158269,0.4,-0.546873841618297));
#11307=CARTESIAN_POINT('Origin',(0.527476652080055,0.4,-0.601471845983182));
#11308=CARTESIAN_POINT('',(0.527476652080055,0.4,-0.601471845983182));
#11309=CARTESIAN_POINT('',(0.527476652080055,0.4,-0.601471845983182));
#11310=CARTESIAN_POINT('',(0.527476652080055,0.4,-0.601471845983182));
#11311=CARTESIAN_POINT('Origin',(0.465982157494242,0.4,-0.650277347673292));
#11312=CARTESIAN_POINT('',(0.465982157494242,0.4,-0.650277347673292));
#11313=CARTESIAN_POINT('',(0.465982157494242,0.4,-0.650277347673292));
#11314=CARTESIAN_POINT('',(0.465982157494242,0.4,-0.650277347673292));
#11315=CARTESIAN_POINT('Origin',(0.4,0.4,-0.692820323027551));
#11316=CARTESIAN_POINT('',(0.4,0.4,-0.692820323027551));
#11317=CARTESIAN_POINT('',(0.4,0.4,-0.692820323027551));
#11318=CARTESIAN_POINT('',(0.4,0.4,-0.692820323027551));
#11319=CARTESIAN_POINT('Origin',(0.330165623843516,0.4,-0.728691059936941));
#11320=CARTESIAN_POINT('',(0.330165623843516,0.4,-0.728691059936941));
#11321=CARTESIAN_POINT('',(0.330165623843516,0.4,-0.728691059936941));
#11322=CARTESIAN_POINT('',(0.330165623843516,0.4,-0.728691059936941));
#11323=CARTESIAN_POINT('Origin',(0.257151572242529,0.4,-0.757544103596084));
#11324=CARTESIAN_POINT('',(0.257151572242529,0.4,-0.757544103596084));
#11325=CARTESIAN_POINT('',(0.257151572242529,0.4,-0.757544103596084));
#11326=CARTESIAN_POINT('',(0.257151572242529,0.4,-0.757544103596084));
#11327=CARTESIAN_POINT('Origin',(0.181661010427499,0.4,-0.779101583421867));
#11328=CARTESIAN_POINT('',(0.181661010427499,0.4,-0.779101583421867));
#11329=CARTESIAN_POINT('',(0.181661010427499,0.4,-0.779101583421867));
#11330=CARTESIAN_POINT('',(0.181661010427499,0.4,-0.779101583421867));
#11331=CARTESIAN_POINT('Origin',(0.104420953776041,0.4,-0.793155889099048));
#11332=CARTESIAN_POINT('',(0.104420953776041,0.4,-0.793155889099048));
#11333=CARTESIAN_POINT('',(0.104420953776041,0.4,-0.793155889099048));
#11334=CARTESIAN_POINT('',(0.104420953776041,0.4,-0.793155889099048));
#11335=CARTESIAN_POINT('Origin',(0.178820883341471,0.4,-1.35827946008212));
#11336=CARTESIAN_POINT('',(0.178820883341471,0.4,-1.35827946008212));
#11337=CARTESIAN_POINT('',(0.178820883341471,0.4,-1.35827946008212));
#11338=CARTESIAN_POINT('',(0.178820883341471,0.4,-1.35827946008212));
#11339=CARTESIAN_POINT('Origin',(0.311094480357091,0.4,-1.33421146160995));
#11340=CARTESIAN_POINT('',(0.311094480357091,0.4,-1.33421146160995));
#11341=CARTESIAN_POINT('',(0.311094480357091,0.4,-1.33421146160995));
#11342=CARTESIAN_POINT('',(0.311094480357092,1.,-1.33421146160995));
#11343=CARTESIAN_POINT('',(0.278026081103186,1.,-1.34022846122799));
#11344=CARTESIAN_POINT('',(0.311094480357091,0.4,-1.33421146160995));
#11345=CARTESIAN_POINT('Origin',(0.440372067465332,0.4,-1.29729427740829));
#11346=CARTESIAN_POINT('',(0.440372067465332,0.4,-1.29729427740829));
#11347=CARTESIAN_POINT('',(0.440372067465332,0.4,-1.29729427740829));
#11348=CARTESIAN_POINT('',(0.440372067465332,1.,-1.29729427740829));
#11349=CARTESIAN_POINT('',(0.408052670688271,1.,-1.30652357345871));
#11350=CARTESIAN_POINT('',(0.440372067465332,0.4,-1.29729427740829));
#11351=CARTESIAN_POINT('Origin',(0.565408630832021,0.4,-1.24788344014201));
#11352=CARTESIAN_POINT('',(0.565408630832021,0.4,-1.24788344014201));
#11353=CARTESIAN_POINT('',(0.565408630832021,0.4,-1.24788344014201));
#11354=CARTESIAN_POINT('',(0.565408630832021,1.,-1.24788344014201));
#11355=CARTESIAN_POINT('',(0.534149489990348,1.,-1.26023614945858));
#11356=CARTESIAN_POINT('',(0.565408630832021,0.4,-1.24788344014201));
#11357=CARTESIAN_POINT('Origin',(0.685,0.4,-1.18645480318468));
#11358=CARTESIAN_POINT('',(0.685,0.4,-1.18645480318468));
#11359=CARTESIAN_POINT('',(0.685,0.4,-1.18645480318468));
#11360=CARTESIAN_POINT('',(0.685,1.,-1.18645480318468));
#11361=CARTESIAN_POINT('',(0.655102157708007,1.,-1.20181196242401));
#11362=CARTESIAN_POINT('',(0.685,0.4,-1.18645480318468));
#11363=CARTESIAN_POINT('Origin',(0.797994444708889,0.4,-1.11359995789051));
#11364=CARTESIAN_POINT('',(0.797994444708889,0.4,-1.11359995789051));
#11365=CARTESIAN_POINT('',(0.797994444708889,0.4,-1.11359995789051));
#11366=CARTESIAN_POINT('',(0.797994444708889,1.,-1.11359995789051));
#11367=CARTESIAN_POINT('',(0.769745833531666,1.,-1.13181366921406));
#11368=CARTESIAN_POINT('',(0.797994444708889,0.4,-1.11359995789051));
#11369=CARTESIAN_POINT('Origin',(0.903303766687094,0.4,-1.0300205362462));
#11370=CARTESIAN_POINT('',(0.903303766687094,0.4,-1.0300205362462));
#11371=CARTESIAN_POINT('',(0.903303766687094,0.4,-1.0300205362462));
#11372=CARTESIAN_POINT('',(0.903303766687094,1.,-1.0300205362462));
#11373=CARTESIAN_POINT('',(0.876976436192544,1.,-1.05091539165728));
#11374=CARTESIAN_POINT('',(0.903303766687094,0.4,-1.0300205362462));
#11375=CARTESIAN_POINT('Origin',(0.999913779596035,0.4,-0.936521453771333));
#11376=CARTESIAN_POINT('',(0.999913779596035,0.4,-0.936521453771333));
#11377=CARTESIAN_POINT('',(0.999913779596035,0.4,-0.936521453771333));
#11378=CARTESIAN_POINT('',(0.999913779596035,1.,-0.936521453771333));
#11379=CARTESIAN_POINT('',(0.9757612763688,1.,-0.959896224390049));
#11380=CARTESIAN_POINT('',(0.999913779596035,0.4,-0.936521453771333));
#11381=CARTESIAN_POINT('Origin',(1.08689407619899,0.4,-0.834003157741947));
#11382=CARTESIAN_POINT('',(1.08689407619899,0.4,-0.834003157741947));
#11383=CARTESIAN_POINT('',(1.08689407619899,0.4,-0.834003157741947));
#11384=CARTESIAN_POINT('',(1.06514900204825,1.,-0.859632731749293));
#11385=CARTESIAN_POINT('',(1.08689407619899,0.4,-0.834003157741947));
#11386=CARTESIAN_POINT('Origin',(0.634682672232988,0.4,-0.487009143206976));
#11387=CARTESIAN_POINT('',(0.634682672232988,0.4,-0.487009143206976));
#11388=CARTESIAN_POINT('Origin',(0.527275906502257,0.4,-0.913268659668847));
#11389=CARTESIAN_POINT('Origin',(0.,1.,0.));
#11390=CARTESIAN_POINT('Origin',(0.,1.,0.));
#11391=CARTESIAN_POINT('Origin',(0.,1.,0.));
#11392=CARTESIAN_POINT('Origin',(0.,1.,0.));
#11393=CARTESIAN_POINT('Origin',(0.,1.,0.));
#11394=CARTESIAN_POINT('Origin',(0.,1.,0.));
#11395=CARTESIAN_POINT('Origin',(0.,1.,0.));
#11396=CARTESIAN_POINT('Origin',(0.,1.,0.));
#11397=CARTESIAN_POINT('Origin',(0.,1.,0.));
#11398=CARTESIAN_POINT('Origin',(0.,1.,0.));
#11399=CARTESIAN_POINT('Origin',(0.,1.,0.));
#11400=CARTESIAN_POINT('Origin',(0.,1.,0.));
#11401=CARTESIAN_POINT('Origin',(0.,1.,0.));
#11402=CARTESIAN_POINT('Origin',(0.,1.,0.));
#11403=CARTESIAN_POINT('Origin',(0.,1.,0.));
#11404=CARTESIAN_POINT('Origin',(0.,1.,0.));
#11405=CARTESIAN_POINT('Origin',(0.,1.,0.));
#11406=CARTESIAN_POINT('',(-0.685,2.05,1.18645480318468));
#11407=CARTESIAN_POINT('Origin',(0.,2.05,0.));
#11408=CARTESIAN_POINT('',(-0.685,1.,1.18645480318468));
#11409=CARTESIAN_POINT('Origin',(0.,2.05,0.));
#12326=UNCERTAINTY_MEASURE_WITH_UNIT(LENGTH_MEASURE(0.001),#12344,
'DISTANCE_ACCURACY_VALUE',
'Maximum model space distance between geometric entities at asserted c
onnectivities');
#12329=UNCERTAINTY_MEASURE_WITH_UNIT(LENGTH_MEASURE(0.001),#12344,
'DISTANCE_ACCURACY_VALUE',
'Maximum model space distance between geometric entities at asserted c
onnectivities');
#12340=(
GEOMETRIC_REPRESENTATION_CONTEXT(3)
GLOBAL_UNCERTAINTY_ASSIGNED_CONTEXT((#12326))
GLOBAL_UNIT_ASSIGNED_CONTEXT((#12344,#12346,#12347))
REPRESENTATION_CONTEXT('','3D')
);
#12343=(
GEOMETRIC_REPRESENTATION_CONTEXT(3)
GLOBAL_UNCERTAINTY_ASSIGNED_CONTEXT((#12329))
GLOBAL_UNIT_ASSIGNED_CONTEXT((#12344,#12346,#12347))
REPRESENTATION_CONTEXT('','3D')
);
#12344=(
LENGTH_UNIT()
NAMED_UNIT(*)
SI_UNIT(.CENTI.,.METRE.)
);
#12346=(
NAMED_UNIT(*)
PLANE_ANGLE_UNIT()
SI_UNIT($,.RADIAN.)
);
#12347=(
NAMED_UNIT(*)
SI_UNIT($,.STERADIAN.)
SOLID_ANGLE_UNIT()
);
#12358=SHAPE_DEFINITION_REPRESENTATION(#12371,#12405);
#12371=PRODUCT_DEFINITION_SHAPE('',$,#12419);
#12405=SHAPE_REPRESENTATION('',(#7735),#12340);
#12408=PRODUCT_DEFINITION_CONTEXT('part definition',#12449,'design');
#12419=PRODUCT_DEFINITION('Hub B','Hub B',#12432,#12408);
#12432=PRODUCT_DEFINITION_FORMATION('',$,#12461);
#12449=APPLICATION_CONTEXT(
'Core Data for Automotive Mechanical Design Process');
#12450=PRODUCT_CONTEXT('part definition',#12449,'mechanical');
#12461=PRODUCT('Hub B','Hub B','Hub B',(#12450));
#12520=COLOUR_RGB('Sky Blue',0.24,0.69,0.87);
#12521=FILL_AREA_STYLE_COLOUR('',#12520);
#12522=FILL_AREA_STYLE('',(#12521));
#12523=SURFACE_STYLE_FILL_AREA(#12522);
#12524=SURFACE_SIDE_STYLE('',(#12523));
#12525=SURFACE_STYLE_USAGE(.BOTH.,#12524);
#12526=PRESENTATION_STYLE_ASSIGNMENT((#12525));
ENDSEC;
END-ISO-10303-21;
